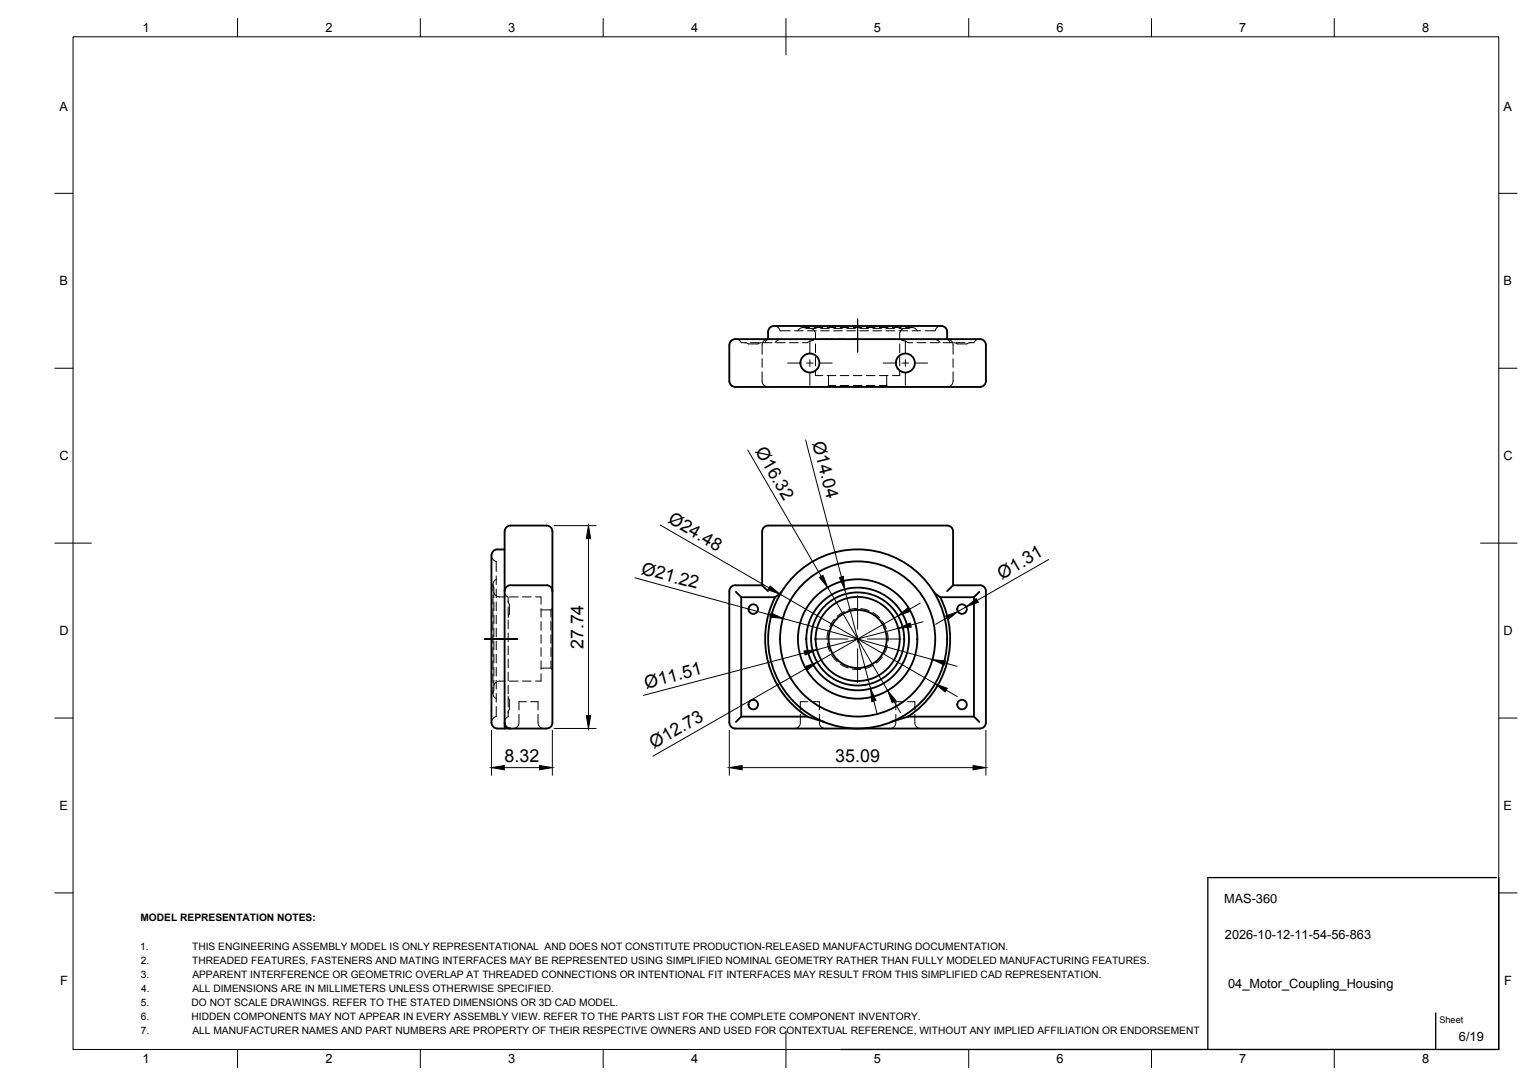
ISO-10303-21;
HEADER;
/* Generated by software containing ST-Developer
 * from STEP Tools, Inc. (www.steptools.com) 
 */

FILE_DESCRIPTION(
/* description */ (''),
/* implementation_level */ '2;1');

FILE_NAME(
/* name */ '04_Motor_Coupling_Housing.step',
/* time_stamp */ '2026-11-04T18:53:29-08:00',
/* author */ (''),
/* organization */ (''),
/* preprocessor_version */ 'ST-DEVELOPER v20.2',
/* originating_system */ 'Autodesk Translation Framework v15.17.0.0',
/* authorisation */ '');

FILE_SCHEMA (('AUTOMOTIVE_DESIGN { 1 0 10303 214 3 1 1 }'));
ENDSEC;

DATA;
#10=MECHANICAL_DESIGN_GEOMETRIC_PRESENTATION_REPRESENTATION('',(#1330),#100031);
#185=SPHERICAL_SURFACE('',#21262,0.800000000000001);
#186=SPHERICAL_SURFACE('',#21266,0.8);
#187=SPHERICAL_SURFACE('',#21275,0.800000000000001);
#188=SPHERICAL_SURFACE('',#21285,0.800000000000001);
#189=SPHERICAL_SURFACE('',#21292,0.800000000000003);
#190=SPHERICAL_SURFACE('',#21298,0.800000000000001);
#191=SPHERICAL_SURFACE('',#21302,0.800000000000001);
#192=SPHERICAL_SURFACE('',#21308,0.800000000000001);
#193=SPHERICAL_SURFACE('',#21315,0.8);
#194=SPHERICAL_SURFACE('',#21323,0.8);
#195=SPHERICAL_SURFACE('',#21330,0.8);
#196=SPHERICAL_SURFACE('',#21334,0.8);
#229=CONICAL_SURFACE('',#21430,4.075,0.785398163397448);
#662=CIRCLE('',#21263,0.800000000000001);
#663=CIRCLE('',#21264,0.800000000000001);
#664=CIRCLE('',#21265,0.800000000000001);
#665=CIRCLE('',#21267,0.800000000000001);
#666=CIRCLE('',#21268,0.8);
#667=CIRCLE('',#21269,0.800000000000001);
#668=CIRCLE('',#21271,0.800000000000001);
#669=CIRCLE('',#21273,0.8);
#670=CIRCLE('',#21276,0.800000000000001);
#671=CIRCLE('',#21277,0.800000000000001);
#672=CIRCLE('',#21278,0.800000000000001);
#673=CIRCLE('',#21280,0.800000000000001);
#674=CIRCLE('',#21286,0.800000000000001);
#675=CIRCLE('',#21287,0.800000000000001);
#676=CIRCLE('',#21288,0.800000000000001);
#677=CIRCLE('',#21291,0.800000000000001);
#678=CIRCLE('',#21293,0.800000000000001);
#679=CIRCLE('',#21294,0.800000000000003);
#680=CIRCLE('',#21295,0.800000000000001);
#681=CIRCLE('',#21299,0.800000000000001);
#682=CIRCLE('',#21300,0.800000000000001);
#683=CIRCLE('',#21301,0.800000000000001);
#684=CIRCLE('',#21303,0.8);
#685=CIRCLE('',#21304,0.800000000000001);
#686=CIRCLE('',#21305,0.800000000000001);
#687=CIRCLE('',#21307,0.8);
#688=CIRCLE('',#21309,0.800000000000001);
#689=CIRCLE('',#21310,0.800000000000001);
#690=CIRCLE('',#21311,0.800000000000001);
#691=CIRCLE('',#21316,0.799999999999998);
#692=CIRCLE('',#21317,0.799999999999997);
#693=CIRCLE('',#21318,0.799999999999999);
#694=CIRCLE('',#21322,0.800000000000001);
#695=CIRCLE('',#21324,0.799999999999999);
#696=CIRCLE('',#21325,0.800000000000001);
#697=CIRCLE('',#21328,0.800000000000001);
#698=CIRCLE('',#21331,0.799999999999999);
#699=CIRCLE('',#21332,12.24);
#700=CIRCLE('',#21333,12.24);
#701=CIRCLE('',#21335,0.800000000000001);
#702=CIRCLE('',#21338,2.1);
#703=CIRCLE('',#21339,2.1);
#704=CIRCLE('',#21350,5.7528);
#705=CIRCLE('',#21351,0.8);
#706=CIRCLE('',#21352,6.3648);
#707=CIRCLE('',#21354,5.7528);
#708=CIRCLE('',#21356,11.44);
#709=CIRCLE('',#21357,0.8);
#710=CIRCLE('',#21358,12.24);
#711=CIRCLE('',#21360,11.3943409947345);
#712=CIRCLE('',#21362,12.24);
#713=CIRCLE('',#21363,12.24);
#714=CIRCLE('',#21364,12.24);
#715=CIRCLE('',#21365,12.24);
#716=CIRCLE('',#21366,12.24);
#717=CIRCLE('',#21367,12.24);
#718=CIRCLE('',#21369,10.608);
#719=CIRCLE('',#21370,0.8);
#720=CIRCLE('',#21372,0.8);
#721=CIRCLE('',#21373,1.3);
#722=CIRCLE('',#21374,1.3);
#723=CIRCLE('',#21376,1.3);
#724=CIRCLE('',#21378,0.8);
#725=CIRCLE('',#21379,1.3);
#726=CIRCLE('',#21380,1.3);
#727=CIRCLE('',#21382,1.3);
#728=CIRCLE('',#21389,12.648);
#729=CIRCLE('',#21391,12.648);
#730=CIRCLE('',#21399,0.6528);
#731=CIRCLE('',#21400,0.8);
#732=CIRCLE('',#21401,1.13703729720046);
#733=CIRCLE('',#21403,1.13703729720046);
#734=CIRCLE('',#21405,0.6528);
#735=CIRCLE('',#21406,0.8);
#736=CIRCLE('',#21408,0.6528);
#737=CIRCLE('',#21409,0.8);
#738=CIRCLE('',#21410,1.13703729720046);
#739=CIRCLE('',#21412,1.13703729720046);
#740=CIRCLE('',#21414,0.6528);
#741=CIRCLE('',#21415,0.8);
#742=CIRCLE('',#21417,8.16);
#743=CIRCLE('',#21418,0.8);
#744=CIRCLE('',#21419,7.0176);
#745=CIRCLE('',#21429,3.975);
#746=CIRCLE('',#21431,3.975);
#747=CIRCLE('',#21432,4.175);
#1237=TOROIDAL_SURFACE('',#21349,6.5528,0.8);
#1238=TOROIDAL_SURFACE('',#21355,11.44,0.8);
#1239=TOROIDAL_SURFACE('',#21368,11.3943409947345,0.8);
#1240=TOROIDAL_SURFACE('',#21371,2.1,0.8);
#1241=TOROIDAL_SURFACE('',#21377,2.1,0.8);
#1242=TOROIDAL_SURFACE('',#21388,11.8802820935674,0.8);
#1243=TOROIDAL_SURFACE('',#21390,11.8802820935674,0.8);
#1244=TOROIDAL_SURFACE('',#21398,1.13703729720046,0.8);
#1245=TOROIDAL_SURFACE('',#21404,1.13703729720046,0.8);
#1246=TOROIDAL_SURFACE('',#21407,1.13703729720046,0.8);
#1247=TOROIDAL_SURFACE('',#21413,1.13703729720046,0.8);
#1248=TOROIDAL_SURFACE('',#21416,7.4416006562771,0.8);
#1294=SHAPE_REPRESENTATION_RELATIONSHIP('SRR','None',#100104,#1312);
#1312=ADVANCED_BREP_SHAPE_REPRESENTATION('',(#1348),#100016);
#1330=STYLED_ITEM('',(#100201),#1348);
#1348=MANIFOLD_SOLID_BREP('Body1',#20120);
#1455=PLANE('',#21336);
#1456=PLANE('',#21337);
#1457=PLANE('',#21340);
#1458=PLANE('',#21342);
#1459=PLANE('',#21343);
#1460=PLANE('',#21348);
#1461=PLANE('',#21359);
#1462=PLANE('',#21392);
#1463=PLANE('',#21402);
#1464=PLANE('',#21411);
#1465=PLANE('',#21420);
#1466=PLANE('',#21421);
#1467=PLANE('',#21422);
#1468=PLANE('',#21423);
#1469=PLANE('',#21424);
#1470=PLANE('',#21425);
#1471=PLANE('',#21426);
#1472=PLANE('',#21427);
#1473=PLANE('',#21428);
#1474=PLANE('',#21434);
#1475=PLANE('',#21435);
#1476=PLANE('',#21436);
#1743=FACE_BOUND('',#6778,.T.);
#1744=FACE_BOUND('',#6779,.T.);
#1745=FACE_BOUND('',#6792,.T.);
#1746=FACE_BOUND('',#6810,.T.);
#1747=FACE_BOUND('',#6811,.T.);
#1748=FACE_BOUND('',#6815,.T.);
#1749=FACE_BOUND('',#6816,.T.);
#1750=FACE_BOUND('',#6820,.T.);
#1751=FACE_BOUND('',#6828,.T.);
#1752=FACE_BOUND('',#6830,.T.);
#1753=FACE_BOUND('',#6834,.T.);
#1893=ELLIPSE('',#21282,1.13137084989848,0.8);
#1894=ELLIPSE('',#21284,1.13137084989848,0.8);
#1895=ELLIPSE('',#21314,1.13137084989848,0.8);
#1896=ELLIPSE('',#21346,1.13137084989848,0.8);
#1897=ELLIPSE('',#21384,1.13137084989848,0.800000000000001);
#1898=ELLIPSE('',#21385,1.13137084989848,0.800000000000001);
#1899=ELLIPSE('',#21394,1.13137084989848,0.8);
#1900=ELLIPSE('',#21396,1.13137084989848,0.799999999999998);
#2530=LINE('',#61146,#3817);
#2531=LINE('',#61147,#3818);
#2532=LINE('',#61152,#3819);
#2533=LINE('',#61153,#3820);
#2534=LINE('',#61155,#3821);
#2535=LINE('',#61156,#3822);
#2536=LINE('',#61167,#3823);
#2537=LINE('',#61168,#3824);
#2538=LINE('',#61171,#3825);
#2539=LINE('',#61173,#3826);
#2540=LINE('',#61177,#3827);
#2541=LINE('',#61179,#3828);
#2542=LINE('',#61189,#3829);
#2543=LINE('',#61190,#3830);
#2544=LINE('',#61195,#3831);
#2545=LINE('',#61196,#3832);
#2546=LINE('',#61205,#3833);
#2547=LINE('',#61206,#3834);
#2548=LINE('',#61208,#3835);
#2549=LINE('',#61209,#3836);
#2550=LINE('',#61228,#3837);
#2551=LINE('',#61229,#3838);
#2552=LINE('',#61238,#3839);
#2553=LINE('',#61239,#3840);
#2554=LINE('',#61242,#3841);
#2555=LINE('',#61244,#3842);
#2556=LINE('',#61254,#3843);
#2557=LINE('',#61255,#3844);
#2558=LINE('',#61257,#3845);
#2559=LINE('',#61258,#3846);
#2560=LINE('',#61263,#3847);
#2561=LINE('',#61264,#3848);
#2562=LINE('',#61270,#3849);
#2563=LINE('',#61271,#3850);
#2564=LINE('',#61275,#3851);
#2565=LINE('',#61276,#3852);
#2566=LINE('',#61278,#3853);
#2567=LINE('',#61279,#3854);
#2568=LINE('',#61389,#3855);
#2569=LINE('',#61391,#3856);
#2570=LINE('',#61397,#3857);
#2571=LINE('',#61399,#3858);
#2572=LINE('',#61403,#3859);
#2573=LINE('',#61406,#3860);
#2574=LINE('',#61409,#3861);
#2575=LINE('',#61411,#3862);
#2576=LINE('',#61412,#3863);
#2577=LINE('',#61414,#3864);
#2578=LINE('',#61424,#3865);
#2579=LINE('',#61436,#3866);
#2580=LINE('',#61459,#3867);
#2581=LINE('',#61469,#3868);
#2582=LINE('',#61474,#3869);
#2583=LINE('',#61478,#3870);
#2584=LINE('',#61496,#3871);
#2585=LINE('',#61497,#3872);
#2586=LINE('',#61516,#3873);
#2587=LINE('',#61517,#3874);
#2588=LINE('',#61558,#3875);
#2589=LINE('',#61560,#3876);
#2590=LINE('',#61561,#3877);
#2591=LINE('',#61565,#3878);
#2592=LINE('',#61568,#3879);
#2593=LINE('',#61571,#3880);
#2594=LINE('',#61619,#3881);
#2595=LINE('',#61622,#3882);
#3817=VECTOR('',#24951,10.);
#3818=VECTOR('',#24952,10.);
#3819=VECTOR('',#24957,10.);
#3820=VECTOR('',#24958,10.);
#3821=VECTOR('',#24961,10.);
#3822=VECTOR('',#24962,10.);
#3823=VECTOR('',#24975,10.);
#3824=VECTOR('',#24976,10.);
#3825=VECTOR('',#24979,10.);
#3826=VECTOR('',#24980,10.);
#3827=VECTOR('',#24985,10.);
#3828=VECTOR('',#24986,10.);
#3829=VECTOR('',#24999,10.);
#3830=VECTOR('',#25000,10.);
#3831=VECTOR('',#25005,10.);
#3832=VECTOR('',#25006,10.);
#3833=VECTOR('',#25017,10.);
#3834=VECTOR('',#25018,10.);
#3835=VECTOR('',#25021,10.);
#3836=VECTOR('',#25022,10.);
#3837=VECTOR('',#25043,10.);
#3838=VECTOR('',#25044,10.);
#3839=VECTOR('',#25055,10.);
#3840=VECTOR('',#25056,10.);
#3841=VECTOR('',#25059,10.);
#3842=VECTOR('',#25060,10.);
#3843=VECTOR('',#25073,10.);
#3844=VECTOR('',#25074,10.);
#3845=VECTOR('',#25077,10.);
#3846=VECTOR('',#25078,10.);
#3847=VECTOR('',#25083,10.);
#3848=VECTOR('',#25084,10.);
#3849=VECTOR('',#25093,10.);
#3850=VECTOR('',#25094,10.);
#3851=VECTOR('',#25099,10.);
#3852=VECTOR('',#25100,10.);
#3853=VECTOR('',#25103,10.);
#3854=VECTOR('',#25104,10.);
#3855=VECTOR('',#25119,10.);
#3856=VECTOR('',#25122,10.);
#3857=VECTOR('',#25129,10.);
#3858=VECTOR('',#25132,10.);
#3859=VECTOR('',#25139,10.);
#3860=VECTOR('',#25142,10.);
#3861=VECTOR('',#25145,10.);
#3862=VECTOR('',#25148,10.);
#3863=VECTOR('',#25149,10.);
#3864=VECTOR('',#25152,10.);
#3865=VECTOR('',#25165,5.7528);
#3866=VECTOR('',#25180,12.24);
#3867=VECTOR('',#25209,1.3);
#3868=VECTOR('',#25222,1.3);
#3869=VECTOR('',#25227,0.8);
#3870=VECTOR('',#25230,10.);
#3871=VECTOR('',#25235,10.);
#3872=VECTOR('',#25236,0.8);
#3873=VECTOR('',#25239,0.8);
#3874=VECTOR('',#25240,10.);
#3875=VECTOR('',#25251,10.);
#3876=VECTOR('',#25252,0.8);
#3877=VECTOR('',#25253,10.);
#3878=VECTOR('',#25258,10.);
#3879=VECTOR('',#25261,10.);
#3880=VECTOR('',#25266,10.);
#3881=VECTOR('',#25335,4.075);
#3882=VECTOR('',#25340,3.975);
#4767=CYLINDRICAL_SURFACE('',#21270,0.8);
#4768=CYLINDRICAL_SURFACE('',#21272,0.8);
#4769=CYLINDRICAL_SURFACE('',#21274,0.8);
#4770=CYLINDRICAL_SURFACE('',#21279,0.8);
#4771=CYLINDRICAL_SURFACE('',#21281,0.8);
#4772=CYLINDRICAL_SURFACE('',#21283,0.8);
#4773=CYLINDRICAL_SURFACE('',#21289,0.8);
#4774=CYLINDRICAL_SURFACE('',#21290,0.8);
#4775=CYLINDRICAL_SURFACE('',#21296,0.8);
#4776=CYLINDRICAL_SURFACE('',#21297,0.8);
#4777=CYLINDRICAL_SURFACE('',#21306,0.8);
#4778=CYLINDRICAL_SURFACE('',#21312,0.8);
#4779=CYLINDRICAL_SURFACE('',#21313,0.8);
#4780=CYLINDRICAL_SURFACE('',#21319,0.8);
#4781=CYLINDRICAL_SURFACE('',#21320,0.8);
#4782=CYLINDRICAL_SURFACE('',#21321,0.8);
#4783=CYLINDRICAL_SURFACE('',#21326,0.8);
#4784=CYLINDRICAL_SURFACE('',#21327,0.8);
#4785=CYLINDRICAL_SURFACE('',#21329,0.8);
#4786=CYLINDRICAL_SURFACE('',#21341,0.8);
#4787=CYLINDRICAL_SURFACE('',#21344,0.8);
#4788=CYLINDRICAL_SURFACE('',#21345,0.8);
#4789=CYLINDRICAL_SURFACE('',#21347,0.8);
#4790=CYLINDRICAL_SURFACE('',#21353,5.7528);
#4791=CYLINDRICAL_SURFACE('',#21361,12.24);
#4792=CYLINDRICAL_SURFACE('',#21375,1.3);
#4793=CYLINDRICAL_SURFACE('',#21381,1.3);
#4794=CYLINDRICAL_SURFACE('',#21383,0.8);
#4795=CYLINDRICAL_SURFACE('',#21386,0.8);
#4796=CYLINDRICAL_SURFACE('',#21387,0.799999999999998);
#4797=CYLINDRICAL_SURFACE('',#21393,0.8);
#4798=CYLINDRICAL_SURFACE('',#21395,0.799999999999998);
#4799=CYLINDRICAL_SURFACE('',#21397,0.8);
#4800=CYLINDRICAL_SURFACE('',#21433,3.975);
#5537=FACE_OUTER_BOUND('',#6743,.T.);
#5538=FACE_OUTER_BOUND('',#6744,.T.);
#5539=FACE_OUTER_BOUND('',#6745,.T.);
#5540=FACE_OUTER_BOUND('',#6746,.T.);
#5541=FACE_OUTER_BOUND('',#6747,.T.);
#5542=FACE_OUTER_BOUND('',#6748,.T.);
#5543=FACE_OUTER_BOUND('',#6749,.T.);
#5544=FACE_OUTER_BOUND('',#6750,.T.);
#5545=FACE_OUTER_BOUND('',#6751,.T.);
#5546=FACE_OUTER_BOUND('',#6752,.T.);
#5547=FACE_OUTER_BOUND('',#6753,.T.);
#5548=FACE_OUTER_BOUND('',#6754,.T.);
#5549=FACE_OUTER_BOUND('',#6755,.T.);
#5550=FACE_OUTER_BOUND('',#6756,.T.);
#5551=FACE_OUTER_BOUND('',#6757,.T.);
#5552=FACE_OUTER_BOUND('',#6758,.T.);
#5553=FACE_OUTER_BOUND('',#6759,.T.);
#5554=FACE_OUTER_BOUND('',#6760,.T.);
#5555=FACE_OUTER_BOUND('',#6761,.T.);
#5556=FACE_OUTER_BOUND('',#6762,.T.);
#5557=FACE_OUTER_BOUND('',#6763,.T.);
#5558=FACE_OUTER_BOUND('',#6764,.T.);
#5559=FACE_OUTER_BOUND('',#6765,.T.);
#5560=FACE_OUTER_BOUND('',#6766,.T.);
#5561=FACE_OUTER_BOUND('',#6767,.T.);
#5562=FACE_OUTER_BOUND('',#6768,.T.);
#5563=FACE_OUTER_BOUND('',#6769,.T.);
#5564=FACE_OUTER_BOUND('',#6770,.T.);
#5565=FACE_OUTER_BOUND('',#6771,.T.);
#5566=FACE_OUTER_BOUND('',#6772,.T.);
#5567=FACE_OUTER_BOUND('',#6773,.T.);
#5568=FACE_OUTER_BOUND('',#6774,.T.);
#5569=FACE_OUTER_BOUND('',#6775,.T.);
#5570=FACE_OUTER_BOUND('',#6776,.T.);
#5571=FACE_OUTER_BOUND('',#6777,.T.);
#5572=FACE_OUTER_BOUND('',#6780,.T.);
#5573=FACE_OUTER_BOUND('',#6781,.T.);
#5574=FACE_OUTER_BOUND('',#6782,.T.);
#5575=FACE_OUTER_BOUND('',#6783,.T.);
#5576=FACE_OUTER_BOUND('',#6784,.T.);
#5577=FACE_OUTER_BOUND('',#6785,.T.);
#5578=FACE_OUTER_BOUND('',#6786,.T.);
#5579=FACE_OUTER_BOUND('',#6787,.T.);
#5580=FACE_OUTER_BOUND('',#6788,.T.);
#5581=FACE_OUTER_BOUND('',#6789,.T.);
#5582=FACE_OUTER_BOUND('',#6790,.T.);
#5583=FACE_OUTER_BOUND('',#6791,.T.);
#5584=FACE_OUTER_BOUND('',#6793,.T.);
#5585=FACE_OUTER_BOUND('',#6794,.T.);
#5586=FACE_OUTER_BOUND('',#6795,.T.);
#5587=FACE_OUTER_BOUND('',#6796,.T.);
#5588=FACE_OUTER_BOUND('',#6797,.T.);
#5589=FACE_OUTER_BOUND('',#6798,.T.);
#5590=FACE_OUTER_BOUND('',#6799,.T.);
#5591=FACE_OUTER_BOUND('',#6800,.T.);
#5592=FACE_OUTER_BOUND('',#6801,.T.);
#5593=FACE_OUTER_BOUND('',#6802,.T.);
#5594=FACE_OUTER_BOUND('',#6803,.T.);
#5595=FACE_OUTER_BOUND('',#6804,.T.);
#5596=FACE_OUTER_BOUND('',#6805,.T.);
#5597=FACE_OUTER_BOUND('',#6806,.T.);
#5598=FACE_OUTER_BOUND('',#6807,.T.);
#5599=FACE_OUTER_BOUND('',#6808,.T.);
#5600=FACE_OUTER_BOUND('',#6809,.T.);
#5601=FACE_OUTER_BOUND('',#6812,.T.);
#5602=FACE_OUTER_BOUND('',#6813,.T.);
#5603=FACE_OUTER_BOUND('',#6814,.T.);
#5604=FACE_OUTER_BOUND('',#6817,.T.);
#5605=FACE_OUTER_BOUND('',#6818,.T.);
#5606=FACE_OUTER_BOUND('',#6819,.T.);
#5607=FACE_OUTER_BOUND('',#6821,.T.);
#5608=FACE_OUTER_BOUND('',#6822,.T.);
#5609=FACE_OUTER_BOUND('',#6823,.T.);
#5610=FACE_OUTER_BOUND('',#6824,.T.);
#5611=FACE_OUTER_BOUND('',#6825,.T.);
#5612=FACE_OUTER_BOUND('',#6826,.T.);
#5613=FACE_OUTER_BOUND('',#6827,.T.);
#5614=FACE_OUTER_BOUND('',#6829,.T.);
#5615=FACE_OUTER_BOUND('',#6831,.T.);
#5616=FACE_OUTER_BOUND('',#6832,.T.);
#5617=FACE_OUTER_BOUND('',#6833,.T.);
#5618=FACE_OUTER_BOUND('',#6835,.T.);
#5619=FACE_OUTER_BOUND('',#6836,.T.);
#6743=EDGE_LOOP('',(#15455,#15456,#15457));
#6744=EDGE_LOOP('',(#15458,#15459,#15460));
#6745=EDGE_LOOP('',(#15461,#15462,#15463,#15464));
#6746=EDGE_LOOP('',(#15465,#15466,#15467,#15468));
#6747=EDGE_LOOP('',(#15469,#15470,#15471,#15472));
#6748=EDGE_LOOP('',(#15473,#15474,#15475));
#6749=EDGE_LOOP('',(#15476,#15477,#15478,#15479));
#6750=EDGE_LOOP('',(#15480,#15481,#15482,#15483));
#6751=EDGE_LOOP('',(#15484,#15485,#15486,#15487));
#6752=EDGE_LOOP('',(#15488,#15489,#15490));
#6753=EDGE_LOOP('',(#15491,#15492,#15493,#15494));
#6754=EDGE_LOOP('',(#15495,#15496,#15497,#15498));
#6755=EDGE_LOOP('',(#15499,#15500,#15501));
#6756=EDGE_LOOP('',(#15502,#15503,#15504,#15505));
#6757=EDGE_LOOP('',(#15506,#15507,#15508,#15509));
#6758=EDGE_LOOP('',(#15510,#15511,#15512));
#6759=EDGE_LOOP('',(#15513,#15514,#15515));
#6760=EDGE_LOOP('',(#15516,#15517,#15518,#15519));
#6761=EDGE_LOOP('',(#15520,#15521,#15522));
#6762=EDGE_LOOP('',(#15523,#15524,#15525,#15526));
#6763=EDGE_LOOP('',(#15527,#15528,#15529,#15530));
#6764=EDGE_LOOP('',(#15531,#15532,#15533));
#6765=EDGE_LOOP('',(#15534,#15535,#15536,#15537));
#6766=EDGE_LOOP('',(#15538,#15539,#15540,#15541));
#6767=EDGE_LOOP('',(#15542,#15543,#15544,#15545));
#6768=EDGE_LOOP('',(#15546,#15547,#15548));
#6769=EDGE_LOOP('',(#15549,#15550,#15551,#15552));
#6770=EDGE_LOOP('',(#15553,#15554,#15555,#15556));
#6771=EDGE_LOOP('',(#15557,#15558,#15559,#15560));
#6772=EDGE_LOOP('',(#15561,#15562,#15563,#15564));
#6773=EDGE_LOOP('',(#15565,#15566,#15567));
#6774=EDGE_LOOP('',(#15568,#15569,#15570,#15571));
#6775=EDGE_LOOP('',(#15572,#15573,#15574));
#6776=EDGE_LOOP('',(#15575,#15576,#15577,#15578));
#6777=EDGE_LOOP('',(#15579,#15580,#15581,#15582,#15583,#15584,#15585));
#6778=EDGE_LOOP('',(#15586));
#6779=EDGE_LOOP('',(#15587));
#6780=EDGE_LOOP('',(#15588,#15589,#15590,#15591));
#6781=EDGE_LOOP('',(#15592,#15593,#15594,#15595));
#6782=EDGE_LOOP('',(#15596,#15597,#15598,#15599));
#6783=EDGE_LOOP('',(#15600,#15601,#15602,#15603));
#6784=EDGE_LOOP('',(#15604,#15605,#15606,#15607));
#6785=EDGE_LOOP('',(#15608,#15609,#15610,#15611));
#6786=EDGE_LOOP('',(#15612,#15613,#15614,#15615));
#6787=EDGE_LOOP('',(#15616,#15617,#15618,#15619));
#6788=EDGE_LOOP('',(#15620,#15621,#15622,#15623));
#6789=EDGE_LOOP('',(#15624,#15625,#15626,#15627));
#6790=EDGE_LOOP('',(#15628,#15629,#15630,#15631));
#6791=EDGE_LOOP('',(#15632));
#6792=EDGE_LOOP('',(#15633));
#6793=EDGE_LOOP('',(#15634,#15635,#15636,#15637,#15638,#15639,#15640,#15641,
#15642,#15643,#15644,#15645,#15646));
#6794=EDGE_LOOP('',(#15647,#15648,#15649,#15650));
#6795=EDGE_LOOP('',(#15651,#15652,#15653,#15654,#15655));
#6796=EDGE_LOOP('',(#15656,#15657,#15658,#15659,#15660));
#6797=EDGE_LOOP('',(#15661,#15662,#15663,#15664,#15665));
#6798=EDGE_LOOP('',(#15666,#15667,#15668,#15669,#15670));
#6799=EDGE_LOOP('',(#15671,#15672,#15673,#15674));
#6800=EDGE_LOOP('',(#15675,#15676,#15677,#15678));
#6801=EDGE_LOOP('',(#15679,#15680,#15681,#15682));
#6802=EDGE_LOOP('',(#15683,#15684,#15685,#15686,#15687));
#6803=EDGE_LOOP('',(#15688,#15689,#15690,#15691));
#6804=EDGE_LOOP('',(#15692,#15693,#15694,#15695,#15696,#15697,#15698,#15699,
#15700,#15701,#15702,#15703,#15704,#15705,#15706,#15707,#15708,#15709));
#6805=EDGE_LOOP('',(#15710,#15711,#15712,#15713));
#6806=EDGE_LOOP('',(#15714,#15715,#15716,#15717));
#6807=EDGE_LOOP('',(#15718,#15719,#15720,#15721));
#6808=EDGE_LOOP('',(#15722,#15723,#15724,#15725));
#6809=EDGE_LOOP('',(#15726,#15727,#15728,#15729));
#6810=EDGE_LOOP('',(#15730));
#6811=EDGE_LOOP('',(#15731));
#6812=EDGE_LOOP('',(#15732,#15733,#15734,#15735));
#6813=EDGE_LOOP('',(#15736,#15737,#15738,#15739));
#6814=EDGE_LOOP('',(#15740,#15741,#15742,#15743));
#6815=EDGE_LOOP('',(#15744));
#6816=EDGE_LOOP('',(#15745));
#6817=EDGE_LOOP('',(#15746,#15747,#15748,#15749));
#6818=EDGE_LOOP('',(#15750,#15751,#15752,#15753));
#6819=EDGE_LOOP('',(#15754));
#6820=EDGE_LOOP('',(#15755));
#6821=EDGE_LOOP('',(#15756));
#6822=EDGE_LOOP('',(#15757));
#6823=EDGE_LOOP('',(#15758));
#6824=EDGE_LOOP('',(#15759));
#6825=EDGE_LOOP('',(#15760));
#6826=EDGE_LOOP('',(#15761));
#6827=EDGE_LOOP('',(#15762));
#6828=EDGE_LOOP('',(#15763));
#6829=EDGE_LOOP('',(#15764));
#6830=EDGE_LOOP('',(#15765));
#6831=EDGE_LOOP('',(#15766,#15767,#15768,#15769));
#6832=EDGE_LOOP('',(#15770,#15771,#15772,#15773));
#6833=EDGE_LOOP('',(#15774,#15775,#15776,#15777,#15778,#15779,#15780,#15781));
#6834=EDGE_LOOP('',(#15782));
#6835=EDGE_LOOP('',(#15783,#15784,#15785,#15786));
#6836=EDGE_LOOP('',(#15787,#15788,#15789,#15790));
#7691=B_SPLINE_CURVE_WITH_KNOTS('',3,(#61321,#61322,#61323,#61324,#61325,
#61326,#61327,#61328),.UNSPECIFIED.,.F.,.F.,(4,1,1,2,4),(0.886448358529016,
0.974711394590892,1.06297443065277,1.3277635388384,1.32899011332275),
 .UNSPECIFIED.);
#7692=B_SPLINE_CURVE_WITH_KNOTS('',3,(#61330,#61331,#61332,#61333),
 .UNSPECIFIED.,.F.,.F.,(4,4),(-0.111726598224603,-0.107341152681297),
 .UNSPECIFIED.);
#7693=B_SPLINE_CURVE_WITH_KNOTS('',3,(#61334,#61335,#61336,#61337,#61338,
#61339,#61340,#61341,#61342,#61343,#61344),.UNSPECIFIED.,.F.,.F.,(4,1,2,
2,2,4),(-0.107341152681297,-0.0558632991123017,0.,0.110861644323643,0.224510220235513,
0.333435958612223),.UNSPECIFIED.);
#7694=B_SPLINE_CURVE_WITH_KNOTS('',3,(#61380,#61381,#61382,#61383,#61384,
#61385),.UNSPECIFIED.,.F.,.F.,(4,2,4),(-0.00122657448435937,0.,0.44131518030938),
 .UNSPECIFIED.);
#7695=B_SPLINE_CURVE_WITH_KNOTS('',3,(#61482,#61483,#61484,#61485,#61486,
#61487,#61488,#61489,#61490,#61491,#61492,#61493,#61494,#61495),
 .UNSPECIFIED.,.F.,.F.,(4,2,2,2,2,2,4),(-4.00267101076923,-3.97980879370467,
-3.86999664917252,-3.77335331431691,-3.71746622872759,-3.69720180919271,
-3.6853266531919),.UNSPECIFIED.);
#7696=B_SPLINE_CURVE_WITH_KNOTS('',3,(#61500,#61501,#61502,#61503,#61504,
#61505,#61506,#61507,#61508,#61509,#61510,#61511,#61512,#61513,#61514,#61515),
 .UNSPECIFIED.,.F.,.F.,(4,2,2,2,2,2,2,4),(-0.827425542979679,-0.826220339571657,
-0.824592036045519,-0.820443574755297,-0.781909027879826,-0.745118942396318,
-0.725073379095867,-0.724859868833872),.UNSPECIFIED.);
#7697=B_SPLINE_CURVE_WITH_KNOTS('',3,(#61522,#61523,#61524,#61525,#61526,
#61527,#61528,#61529,#61530,#61531,#61532,#61533,#61534,#61535),
 .UNSPECIFIED.,.F.,.F.,(4,2,2,2,2,2,4),(0.0275854854772956,0.0545477001455191,
0.147140622467183,0.269392757315554,0.297346368764049,0.310172163976987,
0.314080909465034),.UNSPECIFIED.);
#7698=B_SPLINE_CURVE_WITH_KNOTS('',3,(#61538,#61539,#61540,#61541,#61542,
#61543,#61544,#61545,#61546,#61547,#61548,#61549,#61550,#61551,#61552,#61553,
#61554,#61555),.UNSPECIFIED.,.F.,.F.,(4,2,2,2,2,2,2,2,4),(0.121304483487225,
0.121522867409781,0.122956741161004,0.125266692582563,0.133381651141487,
0.155840009541048,0.198528123526881,0.228063475003939,0.232050075067381),
 .UNSPECIFIED.);
#8819=VERTEX_POINT('',#61129);
#8820=VERTEX_POINT('',#61130);
#8821=VERTEX_POINT('',#61132);
#8822=VERTEX_POINT('',#61136);
#8823=VERTEX_POINT('',#61137);
#8824=VERTEX_POINT('',#61139);
#8825=VERTEX_POINT('',#61143);
#8826=VERTEX_POINT('',#61144);
#8827=VERTEX_POINT('',#61149);
#8828=VERTEX_POINT('',#61150);
#8829=VERTEX_POINT('',#61158);
#8830=VERTEX_POINT('',#61159);
#8831=VERTEX_POINT('',#61161);
#8832=VERTEX_POINT('',#61165);
#8833=VERTEX_POINT('',#61170);
#8834=VERTEX_POINT('',#61172);
#8835=VERTEX_POINT('',#61176);
#8836=VERTEX_POINT('',#61178);
#8837=VERTEX_POINT('',#61182);
#8838=VERTEX_POINT('',#61183);
#8839=VERTEX_POINT('',#61185);
#8840=VERTEX_POINT('',#61192);
#8841=VERTEX_POINT('',#61193);
#8842=VERTEX_POINT('',#61198);
#8843=VERTEX_POINT('',#61199);
#8844=VERTEX_POINT('',#61201);
#8845=VERTEX_POINT('',#61211);
#8846=VERTEX_POINT('',#61212);
#8847=VERTEX_POINT('',#61214);
#8848=VERTEX_POINT('',#61218);
#8849=VERTEX_POINT('',#61219);
#8850=VERTEX_POINT('',#61221);
#8851=VERTEX_POINT('',#61225);
#8852=VERTEX_POINT('',#61226);
#8853=VERTEX_POINT('',#61231);
#8854=VERTEX_POINT('',#61232);
#8855=VERTEX_POINT('',#61234);
#8856=VERTEX_POINT('',#61241);
#8857=VERTEX_POINT('',#61243);
#8858=VERTEX_POINT('',#61247);
#8859=VERTEX_POINT('',#61248);
#8860=VERTEX_POINT('',#61250);
#8861=VERTEX_POINT('',#61260);
#8862=VERTEX_POINT('',#61261);
#8863=VERTEX_POINT('',#61266);
#8864=VERTEX_POINT('',#61273);
#8865=VERTEX_POINT('',#61320);
#8866=VERTEX_POINT('',#61329);
#8867=VERTEX_POINT('',#61377);
#8868=VERTEX_POINT('',#61392);
#8869=VERTEX_POINT('',#61394);
#8870=VERTEX_POINT('',#61405);
#8871=VERTEX_POINT('',#61407);
#8872=VERTEX_POINT('',#61416);
#8873=VERTEX_POINT('',#61418);
#8874=VERTEX_POINT('',#61422);
#8875=VERTEX_POINT('',#61426);
#8876=VERTEX_POINT('',#61428);
#8877=VERTEX_POINT('',#61432);
#8878=VERTEX_POINT('',#61435);
#8879=VERTEX_POINT('',#61437);
#8880=VERTEX_POINT('',#61440);
#8881=VERTEX_POINT('',#61442);
#8882=VERTEX_POINT('',#61444);
#8883=VERTEX_POINT('',#61448);
#8884=VERTEX_POINT('',#61452);
#8885=VERTEX_POINT('',#61454);
#8886=VERTEX_POINT('',#61458);
#8887=VERTEX_POINT('',#61462);
#8888=VERTEX_POINT('',#61464);
#8889=VERTEX_POINT('',#61468);
#8890=VERTEX_POINT('',#61472);
#8891=VERTEX_POINT('',#61473);
#8892=VERTEX_POINT('',#61475);
#8893=VERTEX_POINT('',#61477);
#8894=VERTEX_POINT('',#61481);
#8895=VERTEX_POINT('',#61499);
#8896=VERTEX_POINT('',#61521);
#8897=VERTEX_POINT('',#61536);
#8898=VERTEX_POINT('',#61557);
#8899=VERTEX_POINT('',#61559);
#8900=VERTEX_POINT('',#61563);
#8901=VERTEX_POINT('',#61567);
#8902=VERTEX_POINT('',#61573);
#8903=VERTEX_POINT('',#61575);
#8904=VERTEX_POINT('',#61579);
#8905=VERTEX_POINT('',#61582);
#8906=VERTEX_POINT('',#61586);
#8907=VERTEX_POINT('',#61588);
#8908=VERTEX_POINT('',#61592);
#8909=VERTEX_POINT('',#61595);
#8910=VERTEX_POINT('',#61599);
#8911=VERTEX_POINT('',#61601);
#8912=VERTEX_POINT('',#61613);
#8913=VERTEX_POINT('',#61616);
#8914=VERTEX_POINT('',#61618);
#11202=EDGE_CURVE('',#8819,#8820,#662,.F.);
#11203=EDGE_CURVE('',#8821,#8819,#663,.F.);
#11204=EDGE_CURVE('',#8820,#8821,#664,.F.);
#11205=EDGE_CURVE('',#8822,#8823,#665,.F.);
#11206=EDGE_CURVE('',#8824,#8822,#666,.F.);
#11207=EDGE_CURVE('',#8823,#8824,#667,.F.);
#11208=EDGE_CURVE('',#8825,#8826,#668,.T.);
#11209=EDGE_CURVE('',#8826,#8824,#2530,.T.);
#11210=EDGE_CURVE('',#8822,#8825,#2531,.T.);
#11211=EDGE_CURVE('',#8827,#8828,#669,.T.);
#11212=EDGE_CURVE('',#8828,#8823,#2532,.T.);
#11213=EDGE_CURVE('',#8824,#8827,#2533,.T.);
#11214=EDGE_CURVE('',#8819,#8822,#2534,.T.);
#11215=EDGE_CURVE('',#8823,#8821,#2535,.T.);
#11216=EDGE_CURVE('',#8829,#8830,#670,.F.);
#11217=EDGE_CURVE('',#8831,#8829,#671,.F.);
#11218=EDGE_CURVE('',#8830,#8831,#672,.F.);
#11219=EDGE_CURVE('',#8828,#8832,#673,.T.);
#11220=EDGE_CURVE('',#8832,#8831,#2536,.T.);
#11221=EDGE_CURVE('',#8829,#8828,#2537,.T.);
#11222=EDGE_CURVE('',#8833,#8830,#2538,.T.);
#11223=EDGE_CURVE('',#8831,#8834,#2539,.T.);
#11224=EDGE_CURVE('',#8834,#8833,#1893,.T.);
#11225=EDGE_CURVE('',#8835,#8819,#2540,.T.);
#11226=EDGE_CURVE('',#8820,#8836,#2541,.T.);
#11227=EDGE_CURVE('',#8836,#8835,#1894,.T.);
#11228=EDGE_CURVE('',#8837,#8838,#674,.F.);
#11229=EDGE_CURVE('',#8839,#8837,#675,.F.);
#11230=EDGE_CURVE('',#8838,#8839,#676,.F.);
#11231=EDGE_CURVE('',#8834,#8839,#2542,.T.);
#11232=EDGE_CURVE('',#8837,#8833,#2543,.T.);
#11233=EDGE_CURVE('',#8840,#8841,#677,.T.);
#11234=EDGE_CURVE('',#8841,#8838,#2544,.T.);
#11235=EDGE_CURVE('',#8839,#8840,#2545,.T.);
#11236=EDGE_CURVE('',#8842,#8843,#678,.F.);
#11237=EDGE_CURVE('',#8844,#8842,#679,.F.);
#11238=EDGE_CURVE('',#8843,#8844,#680,.F.);
#11239=EDGE_CURVE('',#8836,#8844,#2546,.T.);
#11240=EDGE_CURVE('',#8842,#8835,#2547,.T.);
#11241=EDGE_CURVE('',#8838,#8843,#2548,.T.);
#11242=EDGE_CURVE('',#8844,#8837,#2549,.T.);
#11243=EDGE_CURVE('',#8845,#8846,#681,.F.);
#11244=EDGE_CURVE('',#8847,#8845,#682,.F.);
#11245=EDGE_CURVE('',#8846,#8847,#683,.F.);
#11246=EDGE_CURVE('',#8848,#8849,#684,.F.);
#11247=EDGE_CURVE('',#8850,#8848,#685,.F.);
#11248=EDGE_CURVE('',#8849,#8850,#686,.F.);
#11249=EDGE_CURVE('',#8851,#8852,#687,.T.);
#11250=EDGE_CURVE('',#8852,#8850,#2550,.T.);
#11251=EDGE_CURVE('',#8848,#8851,#2551,.T.);
#11252=EDGE_CURVE('',#8853,#8854,#688,.F.);
#11253=EDGE_CURVE('',#8855,#8853,#689,.F.);
#11254=EDGE_CURVE('',#8854,#8855,#690,.F.);
#11255=EDGE_CURVE('',#8853,#8849,#2552,.T.);
#11256=EDGE_CURVE('',#8850,#8855,#2553,.T.);
#11257=EDGE_CURVE('',#8856,#8854,#2554,.T.);
#11258=EDGE_CURVE('',#8855,#8857,#2555,.T.);
#11259=EDGE_CURVE('',#8857,#8856,#1895,.T.);
#11260=EDGE_CURVE('',#8858,#8859,#691,.T.);
#11261=EDGE_CURVE('',#8859,#8860,#692,.T.);
#11262=EDGE_CURVE('',#8860,#8858,#693,.T.);
#11263=EDGE_CURVE('',#8858,#8853,#2556,.T.);
#11264=EDGE_CURVE('',#8854,#8859,#2557,.T.);
#11265=EDGE_CURVE('',#8857,#8847,#2558,.T.);
#11266=EDGE_CURVE('',#8845,#8856,#2559,.T.);
#11267=EDGE_CURVE('',#8861,#8862,#694,.T.);
#11268=EDGE_CURVE('',#8862,#8848,#2560,.T.);
#11269=EDGE_CURVE('',#8849,#8861,#2561,.T.);
#11270=EDGE_CURVE('',#8861,#8863,#695,.T.);
#11271=EDGE_CURVE('',#8863,#8862,#696,.T.);
#11272=EDGE_CURVE('',#8843,#8846,#2562,.T.);
#11273=EDGE_CURVE('',#8847,#8842,#2563,.T.);
#11274=EDGE_CURVE('',#8841,#8864,#697,.T.);
#11275=EDGE_CURVE('',#8864,#8845,#2564,.T.);
#11276=EDGE_CURVE('',#8846,#8841,#2565,.T.);
#11277=EDGE_CURVE('',#8830,#8820,#2566,.T.);
#11278=EDGE_CURVE('',#8821,#8829,#2567,.T.);
#11279=EDGE_CURVE('',#8851,#8865,#7691,.T.);
#11280=EDGE_CURVE('',#8865,#8866,#7692,.T.);
#11281=EDGE_CURVE('',#8866,#8852,#7693,.T.);
#11282=EDGE_CURVE('',#8840,#8864,#698,.T.);
#11283=EDGE_CURVE('',#8825,#8867,#699,.T.);
#11284=EDGE_CURVE('',#8867,#8865,#700,.T.);
#11285=EDGE_CURVE('',#8865,#8826,#7694,.T.);
#11286=EDGE_CURVE('',#8827,#8832,#701,.T.);
#11287=EDGE_CURVE('',#8833,#8836,#2568,.T.);
#11288=EDGE_CURVE('',#8827,#8862,#2569,.T.);
#11289=EDGE_CURVE('',#8868,#8868,#702,.T.);
#11290=EDGE_CURVE('',#8869,#8869,#703,.T.);
#11291=EDGE_CURVE('',#8861,#8858,#2570,.T.);
#11292=EDGE_CURVE('',#8860,#8863,#2571,.T.);
#11293=EDGE_CURVE('',#8863,#8832,#2572,.T.);
#11294=EDGE_CURVE('',#8859,#8870,#2573,.T.);
#11295=EDGE_CURVE('',#8870,#8871,#1896,.T.);
#11296=EDGE_CURVE('',#8871,#8860,#2574,.T.);
#11297=EDGE_CURVE('',#8840,#8871,#2575,.T.);
#11298=EDGE_CURVE('',#8870,#8864,#2576,.T.);
#11299=EDGE_CURVE('',#8856,#8870,#2577,.T.);
#11300=EDGE_CURVE('',#8872,#8872,#704,.T.);
#11301=EDGE_CURVE('',#8872,#8873,#705,.T.);
#11302=EDGE_CURVE('',#8873,#8873,#706,.T.);
#11303=EDGE_CURVE('',#8874,#8874,#707,.T.);
#11304=EDGE_CURVE('',#8874,#8872,#2578,.T.);
#11305=EDGE_CURVE('',#8875,#8875,#708,.T.);
#11306=EDGE_CURVE('',#8875,#8876,#709,.T.);
#11307=EDGE_CURVE('',#8876,#8876,#710,.T.);
#11308=EDGE_CURVE('',#8877,#8877,#711,.T.);
#11309=EDGE_CURVE('',#8876,#8878,#2579,.T.);
#11310=EDGE_CURVE('',#8879,#8878,#712,.T.);
#11311=EDGE_CURVE('',#8852,#8879,#713,.T.);
#11312=EDGE_CURVE('',#8880,#8825,#714,.T.);
#11313=EDGE_CURVE('',#8881,#8880,#715,.T.);
#11314=EDGE_CURVE('',#8882,#8881,#716,.T.);
#11315=EDGE_CURVE('',#8878,#8882,#717,.T.);
#11316=EDGE_CURVE('',#8883,#8883,#718,.T.);
#11317=EDGE_CURVE('',#8883,#8877,#719,.T.);
#11318=EDGE_CURVE('',#8869,#8884,#720,.T.);
#11319=EDGE_CURVE('',#8884,#8885,#721,.T.);
#11320=EDGE_CURVE('',#8885,#8884,#722,.T.);
#11321=EDGE_CURVE('',#8885,#8886,#2580,.T.);
#11322=EDGE_CURVE('',#8886,#8886,#723,.T.);
#11323=EDGE_CURVE('',#8868,#8887,#724,.T.);
#11324=EDGE_CURVE('',#8887,#8888,#725,.T.);
#11325=EDGE_CURVE('',#8888,#8887,#726,.T.);
#11326=EDGE_CURVE('',#8888,#8889,#2581,.T.);
#11327=EDGE_CURVE('',#8889,#8889,#727,.T.);
#11328=EDGE_CURVE('',#8890,#8891,#2582,.T.);
#11329=EDGE_CURVE('',#8891,#8892,#1897,.T.);
#11330=EDGE_CURVE('',#8892,#8893,#2583,.T.);
#11331=EDGE_CURVE('',#8893,#8890,#1898,.T.);
#11332=EDGE_CURVE('',#8879,#8894,#7695,.F.);
#11333=EDGE_CURVE('',#8894,#8892,#2584,.T.);
#11334=EDGE_CURVE('',#8891,#8879,#2585,.T.);
#11335=EDGE_CURVE('',#8882,#8895,#7696,.T.);
#11336=EDGE_CURVE('',#8882,#8890,#2586,.T.);
#11337=EDGE_CURVE('',#8893,#8895,#2587,.T.);
#11338=EDGE_CURVE('',#8895,#8894,#728,.T.);
#11339=EDGE_CURVE('',#8880,#8896,#7697,.F.);
#11340=EDGE_CURVE('',#8896,#8897,#729,.T.);
#11341=EDGE_CURVE('',#8881,#8897,#7698,.T.);
#11342=EDGE_CURVE('',#8898,#8881,#2588,.T.);
#11343=EDGE_CURVE('',#8899,#8898,#2589,.T.);
#11344=EDGE_CURVE('',#8880,#8899,#2590,.T.);
#11345=EDGE_CURVE('',#8899,#8900,#1899,.T.);
#11346=EDGE_CURVE('',#8900,#8896,#2591,.T.);
#11347=EDGE_CURVE('',#8897,#8901,#2592,.T.);
#11348=EDGE_CURVE('',#8901,#8898,#1900,.T.);
#11349=EDGE_CURVE('',#8901,#8900,#2593,.T.);
#11350=EDGE_CURVE('',#8902,#8902,#730,.T.);
#11351=EDGE_CURVE('',#8902,#8903,#731,.T.);
#11352=EDGE_CURVE('',#8903,#8903,#732,.T.);
#11353=EDGE_CURVE('',#8904,#8904,#733,.T.);
#11354=EDGE_CURVE('',#8905,#8905,#734,.T.);
#11355=EDGE_CURVE('',#8905,#8904,#735,.T.);
#11356=EDGE_CURVE('',#8906,#8906,#736,.T.);
#11357=EDGE_CURVE('',#8906,#8907,#737,.T.);
#11358=EDGE_CURVE('',#8907,#8907,#738,.T.);
#11359=EDGE_CURVE('',#8908,#8908,#739,.T.);
#11360=EDGE_CURVE('',#8909,#8909,#740,.T.);
#11361=EDGE_CURVE('',#8909,#8908,#741,.T.);
#11362=EDGE_CURVE('',#8910,#8910,#742,.T.);
#11363=EDGE_CURVE('',#8910,#8911,#743,.T.);
#11364=EDGE_CURVE('',#8911,#8911,#744,.T.);
#11365=EDGE_CURVE('',#8912,#8912,#745,.T.);
#11366=EDGE_CURVE('',#8913,#8913,#746,.T.);
#11367=EDGE_CURVE('',#8913,#8914,#2594,.T.);
#11368=EDGE_CURVE('',#8914,#8914,#747,.T.);
#11369=EDGE_CURVE('',#8913,#8912,#2595,.T.);
#15455=ORIENTED_EDGE('',*,*,#11202,.F.);
#15456=ORIENTED_EDGE('',*,*,#11203,.F.);
#15457=ORIENTED_EDGE('',*,*,#11204,.F.);
#15458=ORIENTED_EDGE('',*,*,#11205,.F.);
#15459=ORIENTED_EDGE('',*,*,#11206,.F.);
#15460=ORIENTED_EDGE('',*,*,#11207,.F.);
#15461=ORIENTED_EDGE('',*,*,#11208,.T.);
#15462=ORIENTED_EDGE('',*,*,#11209,.T.);
#15463=ORIENTED_EDGE('',*,*,#11206,.T.);
#15464=ORIENTED_EDGE('',*,*,#11210,.T.);
#15465=ORIENTED_EDGE('',*,*,#11211,.T.);
#15466=ORIENTED_EDGE('',*,*,#11212,.T.);
#15467=ORIENTED_EDGE('',*,*,#11207,.T.);
#15468=ORIENTED_EDGE('',*,*,#11213,.T.);
#15469=ORIENTED_EDGE('',*,*,#11203,.T.);
#15470=ORIENTED_EDGE('',*,*,#11214,.T.);
#15471=ORIENTED_EDGE('',*,*,#11205,.T.);
#15472=ORIENTED_EDGE('',*,*,#11215,.T.);
#15473=ORIENTED_EDGE('',*,*,#11216,.F.);
#15474=ORIENTED_EDGE('',*,*,#11217,.F.);
#15475=ORIENTED_EDGE('',*,*,#11218,.F.);
#15476=ORIENTED_EDGE('',*,*,#11219,.T.);
#15477=ORIENTED_EDGE('',*,*,#11220,.T.);
#15478=ORIENTED_EDGE('',*,*,#11217,.T.);
#15479=ORIENTED_EDGE('',*,*,#11221,.T.);
#15480=ORIENTED_EDGE('',*,*,#11222,.T.);
#15481=ORIENTED_EDGE('',*,*,#11218,.T.);
#15482=ORIENTED_EDGE('',*,*,#11223,.T.);
#15483=ORIENTED_EDGE('',*,*,#11224,.T.);
#15484=ORIENTED_EDGE('',*,*,#11225,.T.);
#15485=ORIENTED_EDGE('',*,*,#11202,.T.);
#15486=ORIENTED_EDGE('',*,*,#11226,.T.);
#15487=ORIENTED_EDGE('',*,*,#11227,.T.);
#15488=ORIENTED_EDGE('',*,*,#11228,.F.);
#15489=ORIENTED_EDGE('',*,*,#11229,.F.);
#15490=ORIENTED_EDGE('',*,*,#11230,.F.);
#15491=ORIENTED_EDGE('',*,*,#11231,.T.);
#15492=ORIENTED_EDGE('',*,*,#11229,.T.);
#15493=ORIENTED_EDGE('',*,*,#11232,.T.);
#15494=ORIENTED_EDGE('',*,*,#11224,.F.);
#15495=ORIENTED_EDGE('',*,*,#11233,.T.);
#15496=ORIENTED_EDGE('',*,*,#11234,.T.);
#15497=ORIENTED_EDGE('',*,*,#11230,.T.);
#15498=ORIENTED_EDGE('',*,*,#11235,.T.);
#15499=ORIENTED_EDGE('',*,*,#11236,.F.);
#15500=ORIENTED_EDGE('',*,*,#11237,.F.);
#15501=ORIENTED_EDGE('',*,*,#11238,.F.);
#15502=ORIENTED_EDGE('',*,*,#11239,.T.);
#15503=ORIENTED_EDGE('',*,*,#11237,.T.);
#15504=ORIENTED_EDGE('',*,*,#11240,.T.);
#15505=ORIENTED_EDGE('',*,*,#11227,.F.);
#15506=ORIENTED_EDGE('',*,*,#11228,.T.);
#15507=ORIENTED_EDGE('',*,*,#11241,.T.);
#15508=ORIENTED_EDGE('',*,*,#11238,.T.);
#15509=ORIENTED_EDGE('',*,*,#11242,.T.);
#15510=ORIENTED_EDGE('',*,*,#11243,.F.);
#15511=ORIENTED_EDGE('',*,*,#11244,.F.);
#15512=ORIENTED_EDGE('',*,*,#11245,.F.);
#15513=ORIENTED_EDGE('',*,*,#11246,.F.);
#15514=ORIENTED_EDGE('',*,*,#11247,.F.);
#15515=ORIENTED_EDGE('',*,*,#11248,.F.);
#15516=ORIENTED_EDGE('',*,*,#11249,.T.);
#15517=ORIENTED_EDGE('',*,*,#11250,.T.);
#15518=ORIENTED_EDGE('',*,*,#11247,.T.);
#15519=ORIENTED_EDGE('',*,*,#11251,.T.);
#15520=ORIENTED_EDGE('',*,*,#11252,.F.);
#15521=ORIENTED_EDGE('',*,*,#11253,.F.);
#15522=ORIENTED_EDGE('',*,*,#11254,.F.);
#15523=ORIENTED_EDGE('',*,*,#11253,.T.);
#15524=ORIENTED_EDGE('',*,*,#11255,.T.);
#15525=ORIENTED_EDGE('',*,*,#11248,.T.);
#15526=ORIENTED_EDGE('',*,*,#11256,.T.);
#15527=ORIENTED_EDGE('',*,*,#11257,.T.);
#15528=ORIENTED_EDGE('',*,*,#11254,.T.);
#15529=ORIENTED_EDGE('',*,*,#11258,.T.);
#15530=ORIENTED_EDGE('',*,*,#11259,.T.);
#15531=ORIENTED_EDGE('',*,*,#11260,.T.);
#15532=ORIENTED_EDGE('',*,*,#11261,.T.);
#15533=ORIENTED_EDGE('',*,*,#11262,.T.);
#15534=ORIENTED_EDGE('',*,*,#11260,.F.);
#15535=ORIENTED_EDGE('',*,*,#11263,.T.);
#15536=ORIENTED_EDGE('',*,*,#11252,.T.);
#15537=ORIENTED_EDGE('',*,*,#11264,.T.);
#15538=ORIENTED_EDGE('',*,*,#11265,.T.);
#15539=ORIENTED_EDGE('',*,*,#11244,.T.);
#15540=ORIENTED_EDGE('',*,*,#11266,.T.);
#15541=ORIENTED_EDGE('',*,*,#11259,.F.);
#15542=ORIENTED_EDGE('',*,*,#11267,.T.);
#15543=ORIENTED_EDGE('',*,*,#11268,.T.);
#15544=ORIENTED_EDGE('',*,*,#11246,.T.);
#15545=ORIENTED_EDGE('',*,*,#11269,.T.);
#15546=ORIENTED_EDGE('',*,*,#11267,.F.);
#15547=ORIENTED_EDGE('',*,*,#11270,.T.);
#15548=ORIENTED_EDGE('',*,*,#11271,.T.);
#15549=ORIENTED_EDGE('',*,*,#11236,.T.);
#15550=ORIENTED_EDGE('',*,*,#11272,.T.);
#15551=ORIENTED_EDGE('',*,*,#11245,.T.);
#15552=ORIENTED_EDGE('',*,*,#11273,.T.);
#15553=ORIENTED_EDGE('',*,*,#11274,.T.);
#15554=ORIENTED_EDGE('',*,*,#11275,.T.);
#15555=ORIENTED_EDGE('',*,*,#11243,.T.);
#15556=ORIENTED_EDGE('',*,*,#11276,.T.);
#15557=ORIENTED_EDGE('',*,*,#11216,.T.);
#15558=ORIENTED_EDGE('',*,*,#11277,.T.);
#15559=ORIENTED_EDGE('',*,*,#11204,.T.);
#15560=ORIENTED_EDGE('',*,*,#11278,.T.);
#15561=ORIENTED_EDGE('',*,*,#11249,.F.);
#15562=ORIENTED_EDGE('',*,*,#11279,.T.);
#15563=ORIENTED_EDGE('',*,*,#11280,.T.);
#15564=ORIENTED_EDGE('',*,*,#11281,.T.);
#15565=ORIENTED_EDGE('',*,*,#11233,.F.);
#15566=ORIENTED_EDGE('',*,*,#11282,.T.);
#15567=ORIENTED_EDGE('',*,*,#11274,.F.);
#15568=ORIENTED_EDGE('',*,*,#11208,.F.);
#15569=ORIENTED_EDGE('',*,*,#11283,.T.);
#15570=ORIENTED_EDGE('',*,*,#11284,.T.);
#15571=ORIENTED_EDGE('',*,*,#11285,.T.);
#15572=ORIENTED_EDGE('',*,*,#11211,.F.);
#15573=ORIENTED_EDGE('',*,*,#11286,.T.);
#15574=ORIENTED_EDGE('',*,*,#11219,.F.);
#15575=ORIENTED_EDGE('',*,*,#11232,.F.);
#15576=ORIENTED_EDGE('',*,*,#11242,.F.);
#15577=ORIENTED_EDGE('',*,*,#11239,.F.);
#15578=ORIENTED_EDGE('',*,*,#11287,.F.);
#15579=ORIENTED_EDGE('',*,*,#11213,.F.);
#15580=ORIENTED_EDGE('',*,*,#11209,.F.);
#15581=ORIENTED_EDGE('',*,*,#11285,.F.);
#15582=ORIENTED_EDGE('',*,*,#11279,.F.);
#15583=ORIENTED_EDGE('',*,*,#11251,.F.);
#15584=ORIENTED_EDGE('',*,*,#11268,.F.);
#15585=ORIENTED_EDGE('',*,*,#11288,.F.);
#15586=ORIENTED_EDGE('',*,*,#11289,.F.);
#15587=ORIENTED_EDGE('',*,*,#11290,.F.);
#15588=ORIENTED_EDGE('',*,*,#11269,.F.);
#15589=ORIENTED_EDGE('',*,*,#11255,.F.);
#15590=ORIENTED_EDGE('',*,*,#11263,.F.);
#15591=ORIENTED_EDGE('',*,*,#11291,.F.);
#15592=ORIENTED_EDGE('',*,*,#11270,.F.);
#15593=ORIENTED_EDGE('',*,*,#11291,.T.);
#15594=ORIENTED_EDGE('',*,*,#11262,.F.);
#15595=ORIENTED_EDGE('',*,*,#11292,.T.);
#15596=ORIENTED_EDGE('',*,*,#11212,.F.);
#15597=ORIENTED_EDGE('',*,*,#11221,.F.);
#15598=ORIENTED_EDGE('',*,*,#11278,.F.);
#15599=ORIENTED_EDGE('',*,*,#11215,.F.);
#15600=ORIENTED_EDGE('',*,*,#11234,.F.);
#15601=ORIENTED_EDGE('',*,*,#11276,.F.);
#15602=ORIENTED_EDGE('',*,*,#11272,.F.);
#15603=ORIENTED_EDGE('',*,*,#11241,.F.);
#15604=ORIENTED_EDGE('',*,*,#11286,.F.);
#15605=ORIENTED_EDGE('',*,*,#11288,.T.);
#15606=ORIENTED_EDGE('',*,*,#11271,.F.);
#15607=ORIENTED_EDGE('',*,*,#11293,.T.);
#15608=ORIENTED_EDGE('',*,*,#11261,.F.);
#15609=ORIENTED_EDGE('',*,*,#11294,.T.);
#15610=ORIENTED_EDGE('',*,*,#11295,.T.);
#15611=ORIENTED_EDGE('',*,*,#11296,.T.);
#15612=ORIENTED_EDGE('',*,*,#11282,.F.);
#15613=ORIENTED_EDGE('',*,*,#11297,.T.);
#15614=ORIENTED_EDGE('',*,*,#11295,.F.);
#15615=ORIENTED_EDGE('',*,*,#11298,.T.);
#15616=ORIENTED_EDGE('',*,*,#11257,.F.);
#15617=ORIENTED_EDGE('',*,*,#11299,.T.);
#15618=ORIENTED_EDGE('',*,*,#11294,.F.);
#15619=ORIENTED_EDGE('',*,*,#11264,.F.);
#15620=ORIENTED_EDGE('',*,*,#11300,.T.);
#15621=ORIENTED_EDGE('',*,*,#11301,.T.);
#15622=ORIENTED_EDGE('',*,*,#11302,.T.);
#15623=ORIENTED_EDGE('',*,*,#11301,.F.);
#15624=ORIENTED_EDGE('',*,*,#11303,.F.);
#15625=ORIENTED_EDGE('',*,*,#11304,.T.);
#15626=ORIENTED_EDGE('',*,*,#11300,.F.);
#15627=ORIENTED_EDGE('',*,*,#11304,.F.);
#15628=ORIENTED_EDGE('',*,*,#11305,.T.);
#15629=ORIENTED_EDGE('',*,*,#11306,.T.);
#15630=ORIENTED_EDGE('',*,*,#11307,.T.);
#15631=ORIENTED_EDGE('',*,*,#11306,.F.);
#15632=ORIENTED_EDGE('',*,*,#11305,.F.);
#15633=ORIENTED_EDGE('',*,*,#11308,.F.);
#15634=ORIENTED_EDGE('',*,*,#11307,.F.);
#15635=ORIENTED_EDGE('',*,*,#11309,.T.);
#15636=ORIENTED_EDGE('',*,*,#11310,.F.);
#15637=ORIENTED_EDGE('',*,*,#11311,.F.);
#15638=ORIENTED_EDGE('',*,*,#11281,.F.);
#15639=ORIENTED_EDGE('',*,*,#11280,.F.);
#15640=ORIENTED_EDGE('',*,*,#11284,.F.);
#15641=ORIENTED_EDGE('',*,*,#11283,.F.);
#15642=ORIENTED_EDGE('',*,*,#11312,.F.);
#15643=ORIENTED_EDGE('',*,*,#11313,.F.);
#15644=ORIENTED_EDGE('',*,*,#11314,.F.);
#15645=ORIENTED_EDGE('',*,*,#11315,.F.);
#15646=ORIENTED_EDGE('',*,*,#11309,.F.);
#15647=ORIENTED_EDGE('',*,*,#11316,.T.);
#15648=ORIENTED_EDGE('',*,*,#11317,.T.);
#15649=ORIENTED_EDGE('',*,*,#11308,.T.);
#15650=ORIENTED_EDGE('',*,*,#11317,.F.);
#15651=ORIENTED_EDGE('',*,*,#11290,.T.);
#15652=ORIENTED_EDGE('',*,*,#11318,.T.);
#15653=ORIENTED_EDGE('',*,*,#11319,.T.);
#15654=ORIENTED_EDGE('',*,*,#11320,.T.);
#15655=ORIENTED_EDGE('',*,*,#11318,.F.);
#15656=ORIENTED_EDGE('',*,*,#11320,.F.);
#15657=ORIENTED_EDGE('',*,*,#11321,.T.);
#15658=ORIENTED_EDGE('',*,*,#11322,.T.);
#15659=ORIENTED_EDGE('',*,*,#11321,.F.);
#15660=ORIENTED_EDGE('',*,*,#11319,.F.);
#15661=ORIENTED_EDGE('',*,*,#11289,.T.);
#15662=ORIENTED_EDGE('',*,*,#11323,.T.);
#15663=ORIENTED_EDGE('',*,*,#11324,.T.);
#15664=ORIENTED_EDGE('',*,*,#11325,.T.);
#15665=ORIENTED_EDGE('',*,*,#11323,.F.);
#15666=ORIENTED_EDGE('',*,*,#11325,.F.);
#15667=ORIENTED_EDGE('',*,*,#11326,.T.);
#15668=ORIENTED_EDGE('',*,*,#11327,.T.);
#15669=ORIENTED_EDGE('',*,*,#11326,.F.);
#15670=ORIENTED_EDGE('',*,*,#11324,.F.);
#15671=ORIENTED_EDGE('',*,*,#11328,.T.);
#15672=ORIENTED_EDGE('',*,*,#11329,.T.);
#15673=ORIENTED_EDGE('',*,*,#11330,.T.);
#15674=ORIENTED_EDGE('',*,*,#11331,.T.);
#15675=ORIENTED_EDGE('',*,*,#11332,.T.);
#15676=ORIENTED_EDGE('',*,*,#11333,.T.);
#15677=ORIENTED_EDGE('',*,*,#11329,.F.);
#15678=ORIENTED_EDGE('',*,*,#11334,.T.);
#15679=ORIENTED_EDGE('',*,*,#11335,.F.);
#15680=ORIENTED_EDGE('',*,*,#11336,.T.);
#15681=ORIENTED_EDGE('',*,*,#11331,.F.);
#15682=ORIENTED_EDGE('',*,*,#11337,.T.);
#15683=ORIENTED_EDGE('',*,*,#11310,.T.);
#15684=ORIENTED_EDGE('',*,*,#11315,.T.);
#15685=ORIENTED_EDGE('',*,*,#11335,.T.);
#15686=ORIENTED_EDGE('',*,*,#11338,.T.);
#15687=ORIENTED_EDGE('',*,*,#11332,.F.);
#15688=ORIENTED_EDGE('',*,*,#11339,.T.);
#15689=ORIENTED_EDGE('',*,*,#11340,.T.);
#15690=ORIENTED_EDGE('',*,*,#11341,.F.);
#15691=ORIENTED_EDGE('',*,*,#11313,.T.);
#15692=ORIENTED_EDGE('',*,*,#11250,.F.);
#15693=ORIENTED_EDGE('',*,*,#11311,.T.);
#15694=ORIENTED_EDGE('',*,*,#11334,.F.);
#15695=ORIENTED_EDGE('',*,*,#11328,.F.);
#15696=ORIENTED_EDGE('',*,*,#11336,.F.);
#15697=ORIENTED_EDGE('',*,*,#11314,.T.);
#15698=ORIENTED_EDGE('',*,*,#11342,.F.);
#15699=ORIENTED_EDGE('',*,*,#11343,.F.);
#15700=ORIENTED_EDGE('',*,*,#11344,.F.);
#15701=ORIENTED_EDGE('',*,*,#11312,.T.);
#15702=ORIENTED_EDGE('',*,*,#11210,.F.);
#15703=ORIENTED_EDGE('',*,*,#11214,.F.);
#15704=ORIENTED_EDGE('',*,*,#11225,.F.);
#15705=ORIENTED_EDGE('',*,*,#11240,.F.);
#15706=ORIENTED_EDGE('',*,*,#11273,.F.);
#15707=ORIENTED_EDGE('',*,*,#11265,.F.);
#15708=ORIENTED_EDGE('',*,*,#11258,.F.);
#15709=ORIENTED_EDGE('',*,*,#11256,.F.);
#15710=ORIENTED_EDGE('',*,*,#11344,.T.);
#15711=ORIENTED_EDGE('',*,*,#11345,.T.);
#15712=ORIENTED_EDGE('',*,*,#11346,.T.);
#15713=ORIENTED_EDGE('',*,*,#11339,.F.);
#15714=ORIENTED_EDGE('',*,*,#11347,.T.);
#15715=ORIENTED_EDGE('',*,*,#11348,.T.);
#15716=ORIENTED_EDGE('',*,*,#11342,.T.);
#15717=ORIENTED_EDGE('',*,*,#11341,.T.);
#15718=ORIENTED_EDGE('',*,*,#11343,.T.);
#15719=ORIENTED_EDGE('',*,*,#11348,.F.);
#15720=ORIENTED_EDGE('',*,*,#11349,.T.);
#15721=ORIENTED_EDGE('',*,*,#11345,.F.);
#15722=ORIENTED_EDGE('',*,*,#11350,.T.);
#15723=ORIENTED_EDGE('',*,*,#11351,.T.);
#15724=ORIENTED_EDGE('',*,*,#11352,.T.);
#15725=ORIENTED_EDGE('',*,*,#11351,.F.);
#15726=ORIENTED_EDGE('',*,*,#11337,.F.);
#15727=ORIENTED_EDGE('',*,*,#11330,.F.);
#15728=ORIENTED_EDGE('',*,*,#11333,.F.);
#15729=ORIENTED_EDGE('',*,*,#11338,.F.);
#15730=ORIENTED_EDGE('',*,*,#11353,.F.);
#15731=ORIENTED_EDGE('',*,*,#11352,.F.);
#15732=ORIENTED_EDGE('',*,*,#11354,.T.);
#15733=ORIENTED_EDGE('',*,*,#11355,.T.);
#15734=ORIENTED_EDGE('',*,*,#11353,.T.);
#15735=ORIENTED_EDGE('',*,*,#11355,.F.);
#15736=ORIENTED_EDGE('',*,*,#11356,.T.);
#15737=ORIENTED_EDGE('',*,*,#11357,.T.);
#15738=ORIENTED_EDGE('',*,*,#11358,.T.);
#15739=ORIENTED_EDGE('',*,*,#11357,.F.);
#15740=ORIENTED_EDGE('',*,*,#11349,.F.);
#15741=ORIENTED_EDGE('',*,*,#11347,.F.);
#15742=ORIENTED_EDGE('',*,*,#11340,.F.);
#15743=ORIENTED_EDGE('',*,*,#11346,.F.);
#15744=ORIENTED_EDGE('',*,*,#11359,.F.);
#15745=ORIENTED_EDGE('',*,*,#11358,.F.);
#15746=ORIENTED_EDGE('',*,*,#11360,.T.);
#15747=ORIENTED_EDGE('',*,*,#11361,.T.);
#15748=ORIENTED_EDGE('',*,*,#11359,.T.);
#15749=ORIENTED_EDGE('',*,*,#11361,.F.);
#15750=ORIENTED_EDGE('',*,*,#11362,.T.);
#15751=ORIENTED_EDGE('',*,*,#11363,.T.);
#15752=ORIENTED_EDGE('',*,*,#11364,.T.);
#15753=ORIENTED_EDGE('',*,*,#11363,.F.);
#15754=ORIENTED_EDGE('',*,*,#11364,.F.);
#15755=ORIENTED_EDGE('',*,*,#11302,.F.);
#15756=ORIENTED_EDGE('',*,*,#11360,.F.);
#15757=ORIENTED_EDGE('',*,*,#11356,.F.);
#15758=ORIENTED_EDGE('',*,*,#11354,.F.);
#15759=ORIENTED_EDGE('',*,*,#11350,.F.);
#15760=ORIENTED_EDGE('',*,*,#11327,.F.);
#15761=ORIENTED_EDGE('',*,*,#11322,.F.);
#15762=ORIENTED_EDGE('',*,*,#11316,.F.);
#15763=ORIENTED_EDGE('',*,*,#11362,.F.);
#15764=ORIENTED_EDGE('',*,*,#11303,.T.);
#15765=ORIENTED_EDGE('',*,*,#11365,.F.);
#15766=ORIENTED_EDGE('',*,*,#11366,.T.);
#15767=ORIENTED_EDGE('',*,*,#11367,.T.);
#15768=ORIENTED_EDGE('',*,*,#11368,.T.);
#15769=ORIENTED_EDGE('',*,*,#11367,.F.);
#15770=ORIENTED_EDGE('',*,*,#11366,.F.);
#15771=ORIENTED_EDGE('',*,*,#11369,.T.);
#15772=ORIENTED_EDGE('',*,*,#11365,.T.);
#15773=ORIENTED_EDGE('',*,*,#11369,.F.);
#15774=ORIENTED_EDGE('',*,*,#11220,.F.);
#15775=ORIENTED_EDGE('',*,*,#11293,.F.);
#15776=ORIENTED_EDGE('',*,*,#11292,.F.);
#15777=ORIENTED_EDGE('',*,*,#11296,.F.);
#15778=ORIENTED_EDGE('',*,*,#11297,.F.);
#15779=ORIENTED_EDGE('',*,*,#11235,.F.);
#15780=ORIENTED_EDGE('',*,*,#11231,.F.);
#15781=ORIENTED_EDGE('',*,*,#11223,.F.);
#15782=ORIENTED_EDGE('',*,*,#11368,.F.);
#15783=ORIENTED_EDGE('',*,*,#11275,.F.);
#15784=ORIENTED_EDGE('',*,*,#11298,.F.);
#15785=ORIENTED_EDGE('',*,*,#11299,.F.);
#15786=ORIENTED_EDGE('',*,*,#11266,.F.);
#15787=ORIENTED_EDGE('',*,*,#11222,.F.);
#15788=ORIENTED_EDGE('',*,*,#11287,.T.);
#15789=ORIENTED_EDGE('',*,*,#11226,.F.);
#15790=ORIENTED_EDGE('',*,*,#11277,.F.);
#18931=B_SPLINE_SURFACE_WITH_KNOTS('',3,3,((#61280,#61281,#61282,#61283,
#61284,#61285,#61286,#61287),(#61288,#61289,#61290,#61291,#61292,#61293,
#61294,#61295),(#61296,#61297,#61298,#61299,#61300,#61301,#61302,#61303),
(#61304,#61305,#61306,#61307,#61308,#61309,#61310,#61311),(#61312,#61313,
#61314,#61315,#61316,#61317,#61318,#61319)),.UNSPECIFIED.,.F.,.F.,.F.,(4,
1,4),(4,2,1,1,4),(-0.00184352937430784,0.571428571428571,1.),(-1.32899011332275,
-1.3277635388384,-1.06297443065277,-0.974711394590892,-0.884839152512737),
 .UNSPECIFIED.);
#18932=B_SPLINE_SURFACE_WITH_KNOTS('',3,3,((#61347,#61348,#61349,#61350,
#61351,#61352),(#61353,#61354,#61355,#61356,#61357,#61358),(#61359,#61360,
#61361,#61362,#61363,#61364),(#61365,#61366,#61367,#61368,#61369,#61370),
(#61371,#61372,#61373,#61374,#61375,#61376)),.UNSPECIFIED.,.F.,.F.,.F.,
(4,1,4),(4,2,4),(-0.0048972902445563,0.571428571428571,1.),(-0.446212470553937,
0.,0.00122657448435937),.UNSPECIFIED.);
#19471=ADVANCED_FACE('',(#5537),#185,.T.);
#19472=ADVANCED_FACE('',(#5538),#186,.T.);
#19473=ADVANCED_FACE('',(#5539),#4767,.T.);
#19474=ADVANCED_FACE('',(#5540),#4768,.T.);
#19475=ADVANCED_FACE('',(#5541),#4769,.T.);
#19476=ADVANCED_FACE('',(#5542),#187,.T.);
#19477=ADVANCED_FACE('',(#5543),#4770,.T.);
#19478=ADVANCED_FACE('',(#5544),#4771,.T.);
#19479=ADVANCED_FACE('',(#5545),#4772,.T.);
#19480=ADVANCED_FACE('',(#5546),#188,.T.);
#19481=ADVANCED_FACE('',(#5547),#4773,.T.);
#19482=ADVANCED_FACE('',(#5548),#4774,.T.);
#19483=ADVANCED_FACE('',(#5549),#189,.T.);
#19484=ADVANCED_FACE('',(#5550),#4775,.T.);
#19485=ADVANCED_FACE('',(#5551),#4776,.T.);
#19486=ADVANCED_FACE('',(#5552),#190,.T.);
#19487=ADVANCED_FACE('',(#5553),#191,.T.);
#19488=ADVANCED_FACE('',(#5554),#4777,.T.);
#19489=ADVANCED_FACE('',(#5555),#192,.T.);
#19490=ADVANCED_FACE('',(#5556),#4778,.T.);
#19491=ADVANCED_FACE('',(#5557),#4779,.T.);
#19492=ADVANCED_FACE('',(#5558),#193,.T.);
#19493=ADVANCED_FACE('',(#5559),#4780,.T.);
#19494=ADVANCED_FACE('',(#5560),#4781,.T.);
#19495=ADVANCED_FACE('',(#5561),#4782,.T.);
#19496=ADVANCED_FACE('',(#5562),#194,.T.);
#19497=ADVANCED_FACE('',(#5563),#4783,.T.);
#19498=ADVANCED_FACE('',(#5564),#4784,.T.);
#19499=ADVANCED_FACE('',(#5565),#4785,.T.);
#19500=ADVANCED_FACE('',(#5566),#18931,.F.);
#19501=ADVANCED_FACE('',(#5567),#195,.T.);
#19502=ADVANCED_FACE('',(#5568),#18932,.F.);
#19503=ADVANCED_FACE('',(#5569),#196,.T.);
#19504=ADVANCED_FACE('',(#5570),#1455,.T.);
#19505=ADVANCED_FACE('',(#5571,#1743,#1744),#1456,.F.);
#19506=ADVANCED_FACE('',(#5572),#1457,.T.);
#19507=ADVANCED_FACE('',(#5573),#4786,.T.);
#19508=ADVANCED_FACE('',(#5574),#1458,.T.);
#19509=ADVANCED_FACE('',(#5575),#1459,.T.);
#19510=ADVANCED_FACE('',(#5576),#4787,.T.);
#19511=ADVANCED_FACE('',(#5577),#4788,.T.);
#19512=ADVANCED_FACE('',(#5578),#4789,.T.);
#19513=ADVANCED_FACE('',(#5579),#1460,.T.);
#19514=ADVANCED_FACE('',(#5580),#1237,.T.);
#19515=ADVANCED_FACE('',(#5581),#4790,.F.);
#19516=ADVANCED_FACE('',(#5582),#1238,.T.);
#19517=ADVANCED_FACE('',(#5583,#1745),#1461,.T.);
#19518=ADVANCED_FACE('',(#5584),#4791,.T.);
#19519=ADVANCED_FACE('',(#5585),#1239,.T.);
#19520=ADVANCED_FACE('',(#5586),#1240,.T.);
#19521=ADVANCED_FACE('',(#5587),#4792,.F.);
#19522=ADVANCED_FACE('',(#5588),#1241,.T.);
#19523=ADVANCED_FACE('',(#5589),#4793,.F.);
#19524=ADVANCED_FACE('',(#5590),#4794,.T.);
#19525=ADVANCED_FACE('',(#5591),#4795,.T.);
#19526=ADVANCED_FACE('',(#5592),#4796,.T.);
#19527=ADVANCED_FACE('',(#5593),#1242,.T.);
#19528=ADVANCED_FACE('',(#5594),#1243,.T.);
#19529=ADVANCED_FACE('',(#5595),#1462,.T.);
#19530=ADVANCED_FACE('',(#5596),#4797,.T.);
#19531=ADVANCED_FACE('',(#5597),#4798,.T.);
#19532=ADVANCED_FACE('',(#5598),#4799,.T.);
#19533=ADVANCED_FACE('',(#5599),#1244,.T.);
#19534=ADVANCED_FACE('',(#5600,#1746,#1747),#1463,.T.);
#19535=ADVANCED_FACE('',(#5601),#1245,.T.);
#19536=ADVANCED_FACE('',(#5602),#1246,.T.);
#19537=ADVANCED_FACE('',(#5603,#1748,#1749),#1464,.T.);
#19538=ADVANCED_FACE('',(#5604),#1247,.T.);
#19539=ADVANCED_FACE('',(#5605),#1248,.T.);
#19540=ADVANCED_FACE('',(#5606,#1750),#1465,.T.);
#19541=ADVANCED_FACE('',(#5607),#1466,.T.);
#19542=ADVANCED_FACE('',(#5608),#1467,.T.);
#19543=ADVANCED_FACE('',(#5609),#1468,.T.);
#19544=ADVANCED_FACE('',(#5610),#1469,.T.);
#19545=ADVANCED_FACE('',(#5611),#1470,.F.);
#19546=ADVANCED_FACE('',(#5612),#1471,.F.);
#19547=ADVANCED_FACE('',(#5613,#1751),#1472,.T.);
#19548=ADVANCED_FACE('',(#5614,#1752),#1473,.T.);
#19549=ADVANCED_FACE('',(#5615),#229,.F.);
#19550=ADVANCED_FACE('',(#5616),#4800,.F.);
#19551=ADVANCED_FACE('',(#5617,#1753),#1474,.T.);
#19552=ADVANCED_FACE('',(#5618),#1475,.T.);
#19553=ADVANCED_FACE('',(#5619),#1476,.T.);
#20120=CLOSED_SHELL('',(#19471,#19472,#19473,#19474,#19475,#19476,#19477,
#19478,#19479,#19480,#19481,#19482,#19483,#19484,#19485,#19486,#19487,#19488,
#19489,#19490,#19491,#19492,#19493,#19494,#19495,#19496,#19497,#19498,#19499,
#19500,#19501,#19502,#19503,#19504,#19505,#19506,#19507,#19508,#19509,#19510,
#19511,#19512,#19513,#19514,#19515,#19516,#19517,#19518,#19519,#19520,#19521,
#19522,#19523,#19524,#19525,#19526,#19527,#19528,#19529,#19530,#19531,#19532,
#19533,#19534,#19535,#19536,#19537,#19538,#19539,#19540,#19541,#19542,#19543,
#19544,#19545,#19546,#19547,#19548,#19549,#19550,#19551,#19552,#19553));
#21261=AXIS2_PLACEMENT_3D('',#61127,#24929,#24930);
#21262=AXIS2_PLACEMENT_3D('',#61128,#24931,#24932);
#21263=AXIS2_PLACEMENT_3D('',#61131,#24933,#24934);
#21264=AXIS2_PLACEMENT_3D('',#61133,#24935,#24936);
#21265=AXIS2_PLACEMENT_3D('',#61134,#24937,#24938);
#21266=AXIS2_PLACEMENT_3D('',#61135,#24939,#24940);
#21267=AXIS2_PLACEMENT_3D('',#61138,#24941,#24942);
#21268=AXIS2_PLACEMENT_3D('',#61140,#24943,#24944);
#21269=AXIS2_PLACEMENT_3D('',#61141,#24945,#24946);
#21270=AXIS2_PLACEMENT_3D('',#61142,#24947,#24948);
#21271=AXIS2_PLACEMENT_3D('',#61145,#24949,#24950);
#21272=AXIS2_PLACEMENT_3D('',#61148,#24953,#24954);
#21273=AXIS2_PLACEMENT_3D('',#61151,#24955,#24956);
#21274=AXIS2_PLACEMENT_3D('',#61154,#24959,#24960);
#21275=AXIS2_PLACEMENT_3D('',#61157,#24963,#24964);
#21276=AXIS2_PLACEMENT_3D('',#61160,#24965,#24966);
#21277=AXIS2_PLACEMENT_3D('',#61162,#24967,#24968);
#21278=AXIS2_PLACEMENT_3D('',#61163,#24969,#24970);
#21279=AXIS2_PLACEMENT_3D('',#61164,#24971,#24972);
#21280=AXIS2_PLACEMENT_3D('',#61166,#24973,#24974);
#21281=AXIS2_PLACEMENT_3D('',#61169,#24977,#24978);
#21282=AXIS2_PLACEMENT_3D('',#61174,#24981,#24982);
#21283=AXIS2_PLACEMENT_3D('',#61175,#24983,#24984);
#21284=AXIS2_PLACEMENT_3D('',#61180,#24987,#24988);
#21285=AXIS2_PLACEMENT_3D('',#61181,#24989,#24990);
#21286=AXIS2_PLACEMENT_3D('',#61184,#24991,#24992);
#21287=AXIS2_PLACEMENT_3D('',#61186,#24993,#24994);
#21288=AXIS2_PLACEMENT_3D('',#61187,#24995,#24996);
#21289=AXIS2_PLACEMENT_3D('',#61188,#24997,#24998);
#21290=AXIS2_PLACEMENT_3D('',#61191,#25001,#25002);
#21291=AXIS2_PLACEMENT_3D('',#61194,#25003,#25004);
#21292=AXIS2_PLACEMENT_3D('',#61197,#25007,#25008);
#21293=AXIS2_PLACEMENT_3D('',#61200,#25009,#25010);
#21294=AXIS2_PLACEMENT_3D('',#61202,#25011,#25012);
#21295=AXIS2_PLACEMENT_3D('',#61203,#25013,#25014);
#21296=AXIS2_PLACEMENT_3D('',#61204,#25015,#25016);
#21297=AXIS2_PLACEMENT_3D('',#61207,#25019,#25020);
#21298=AXIS2_PLACEMENT_3D('',#61210,#25023,#25024);
#21299=AXIS2_PLACEMENT_3D('',#61213,#25025,#25026);
#21300=AXIS2_PLACEMENT_3D('',#61215,#25027,#25028);
#21301=AXIS2_PLACEMENT_3D('',#61216,#25029,#25030);
#21302=AXIS2_PLACEMENT_3D('',#61217,#25031,#25032);
#21303=AXIS2_PLACEMENT_3D('',#61220,#25033,#25034);
#21304=AXIS2_PLACEMENT_3D('',#61222,#25035,#25036);
#21305=AXIS2_PLACEMENT_3D('',#61223,#25037,#25038);
#21306=AXIS2_PLACEMENT_3D('',#61224,#25039,#25040);
#21307=AXIS2_PLACEMENT_3D('',#61227,#25041,#25042);
#21308=AXIS2_PLACEMENT_3D('',#61230,#25045,#25046);
#21309=AXIS2_PLACEMENT_3D('',#61233,#25047,#25048);
#21310=AXIS2_PLACEMENT_3D('',#61235,#25049,#25050);
#21311=AXIS2_PLACEMENT_3D('',#61236,#25051,#25052);
#21312=AXIS2_PLACEMENT_3D('',#61237,#25053,#25054);
#21313=AXIS2_PLACEMENT_3D('',#61240,#25057,#25058);
#21314=AXIS2_PLACEMENT_3D('',#61245,#25061,#25062);
#21315=AXIS2_PLACEMENT_3D('',#61246,#25063,#25064);
#21316=AXIS2_PLACEMENT_3D('',#61249,#25065,#25066);
#21317=AXIS2_PLACEMENT_3D('',#61251,#25067,#25068);
#21318=AXIS2_PLACEMENT_3D('',#61252,#25069,#25070);
#21319=AXIS2_PLACEMENT_3D('',#61253,#25071,#25072);
#21320=AXIS2_PLACEMENT_3D('',#61256,#25075,#25076);
#21321=AXIS2_PLACEMENT_3D('',#61259,#25079,#25080);
#21322=AXIS2_PLACEMENT_3D('',#61262,#25081,#25082);
#21323=AXIS2_PLACEMENT_3D('',#61265,#25085,#25086);
#21324=AXIS2_PLACEMENT_3D('',#61267,#25087,#25088);
#21325=AXIS2_PLACEMENT_3D('',#61268,#25089,#25090);
#21326=AXIS2_PLACEMENT_3D('',#61269,#25091,#25092);
#21327=AXIS2_PLACEMENT_3D('',#61272,#25095,#25096);
#21328=AXIS2_PLACEMENT_3D('',#61274,#25097,#25098);
#21329=AXIS2_PLACEMENT_3D('',#61277,#25101,#25102);
#21330=AXIS2_PLACEMENT_3D('',#61345,#25105,#25106);
#21331=AXIS2_PLACEMENT_3D('',#61346,#25107,#25108);
#21332=AXIS2_PLACEMENT_3D('',#61378,#25109,#25110);
#21333=AXIS2_PLACEMENT_3D('',#61379,#25111,#25112);
#21334=AXIS2_PLACEMENT_3D('',#61386,#25113,#25114);
#21335=AXIS2_PLACEMENT_3D('',#61387,#25115,#25116);
#21336=AXIS2_PLACEMENT_3D('',#61388,#25117,#25118);
#21337=AXIS2_PLACEMENT_3D('',#61390,#25120,#25121);
#21338=AXIS2_PLACEMENT_3D('',#61393,#25123,#25124);
#21339=AXIS2_PLACEMENT_3D('',#61395,#25125,#25126);
#21340=AXIS2_PLACEMENT_3D('',#61396,#25127,#25128);
#21341=AXIS2_PLACEMENT_3D('',#61398,#25130,#25131);
#21342=AXIS2_PLACEMENT_3D('',#61400,#25133,#25134);
#21343=AXIS2_PLACEMENT_3D('',#61401,#25135,#25136);
#21344=AXIS2_PLACEMENT_3D('',#61402,#25137,#25138);
#21345=AXIS2_PLACEMENT_3D('',#61404,#25140,#25141);
#21346=AXIS2_PLACEMENT_3D('',#61408,#25143,#25144);
#21347=AXIS2_PLACEMENT_3D('',#61410,#25146,#25147);
#21348=AXIS2_PLACEMENT_3D('',#61413,#25150,#25151);
#21349=AXIS2_PLACEMENT_3D('',#61415,#25153,#25154);
#21350=AXIS2_PLACEMENT_3D('',#61417,#25155,#25156);
#21351=AXIS2_PLACEMENT_3D('',#61419,#25157,#25158);
#21352=AXIS2_PLACEMENT_3D('',#61420,#25159,#25160);
#21353=AXIS2_PLACEMENT_3D('',#61421,#25161,#25162);
#21354=AXIS2_PLACEMENT_3D('',#61423,#25163,#25164);
#21355=AXIS2_PLACEMENT_3D('',#61425,#25166,#25167);
#21356=AXIS2_PLACEMENT_3D('',#61427,#25168,#25169);
#21357=AXIS2_PLACEMENT_3D('',#61429,#25170,#25171);
#21358=AXIS2_PLACEMENT_3D('',#61430,#25172,#25173);
#21359=AXIS2_PLACEMENT_3D('',#61431,#25174,#25175);
#21360=AXIS2_PLACEMENT_3D('',#61433,#25176,#25177);
#21361=AXIS2_PLACEMENT_3D('',#61434,#25178,#25179);
#21362=AXIS2_PLACEMENT_3D('',#61438,#25181,#25182);
#21363=AXIS2_PLACEMENT_3D('',#61439,#25183,#25184);
#21364=AXIS2_PLACEMENT_3D('',#61441,#25185,#25186);
#21365=AXIS2_PLACEMENT_3D('',#61443,#25187,#25188);
#21366=AXIS2_PLACEMENT_3D('',#61445,#25189,#25190);
#21367=AXIS2_PLACEMENT_3D('',#61446,#25191,#25192);
#21368=AXIS2_PLACEMENT_3D('',#61447,#25193,#25194);
#21369=AXIS2_PLACEMENT_3D('',#61449,#25195,#25196);
#21370=AXIS2_PLACEMENT_3D('',#61450,#25197,#25198);
#21371=AXIS2_PLACEMENT_3D('',#61451,#25199,#25200);
#21372=AXIS2_PLACEMENT_3D('',#61453,#25201,#25202);
#21373=AXIS2_PLACEMENT_3D('',#61455,#25203,#25204);
#21374=AXIS2_PLACEMENT_3D('',#61456,#25205,#25206);
#21375=AXIS2_PLACEMENT_3D('',#61457,#25207,#25208);
#21376=AXIS2_PLACEMENT_3D('',#61460,#25210,#25211);
#21377=AXIS2_PLACEMENT_3D('',#61461,#25212,#25213);
#21378=AXIS2_PLACEMENT_3D('',#61463,#25214,#25215);
#21379=AXIS2_PLACEMENT_3D('',#61465,#25216,#25217);
#21380=AXIS2_PLACEMENT_3D('',#61466,#25218,#25219);
#21381=AXIS2_PLACEMENT_3D('',#61467,#25220,#25221);
#21382=AXIS2_PLACEMENT_3D('',#61470,#25223,#25224);
#21383=AXIS2_PLACEMENT_3D('',#61471,#25225,#25226);
#21384=AXIS2_PLACEMENT_3D('',#61476,#25228,#25229);
#21385=AXIS2_PLACEMENT_3D('',#61479,#25231,#25232);
#21386=AXIS2_PLACEMENT_3D('',#61480,#25233,#25234);
#21387=AXIS2_PLACEMENT_3D('',#61498,#25237,#25238);
#21388=AXIS2_PLACEMENT_3D('',#61518,#25241,#25242);
#21389=AXIS2_PLACEMENT_3D('',#61519,#25243,#25244);
#21390=AXIS2_PLACEMENT_3D('',#61520,#25245,#25246);
#21391=AXIS2_PLACEMENT_3D('',#61537,#25247,#25248);
#21392=AXIS2_PLACEMENT_3D('',#61556,#25249,#25250);
#21393=AXIS2_PLACEMENT_3D('',#61562,#25254,#25255);
#21394=AXIS2_PLACEMENT_3D('',#61564,#25256,#25257);
#21395=AXIS2_PLACEMENT_3D('',#61566,#25259,#25260);
#21396=AXIS2_PLACEMENT_3D('',#61569,#25262,#25263);
#21397=AXIS2_PLACEMENT_3D('',#61570,#25264,#25265);
#21398=AXIS2_PLACEMENT_3D('',#61572,#25267,#25268);
#21399=AXIS2_PLACEMENT_3D('',#61574,#25269,#25270);
#21400=AXIS2_PLACEMENT_3D('',#61576,#25271,#25272);
#21401=AXIS2_PLACEMENT_3D('',#61577,#25273,#25274);
#21402=AXIS2_PLACEMENT_3D('',#61578,#25275,#25276);
#21403=AXIS2_PLACEMENT_3D('',#61580,#25277,#25278);
#21404=AXIS2_PLACEMENT_3D('',#61581,#25279,#25280);
#21405=AXIS2_PLACEMENT_3D('',#61583,#25281,#25282);
#21406=AXIS2_PLACEMENT_3D('',#61584,#25283,#25284);
#21407=AXIS2_PLACEMENT_3D('',#61585,#25285,#25286);
#21408=AXIS2_PLACEMENT_3D('',#61587,#25287,#25288);
#21409=AXIS2_PLACEMENT_3D('',#61589,#25289,#25290);
#21410=AXIS2_PLACEMENT_3D('',#61590,#25291,#25292);
#21411=AXIS2_PLACEMENT_3D('',#61591,#25293,#25294);
#21412=AXIS2_PLACEMENT_3D('',#61593,#25295,#25296);
#21413=AXIS2_PLACEMENT_3D('',#61594,#25297,#25298);
#21414=AXIS2_PLACEMENT_3D('',#61596,#25299,#25300);
#21415=AXIS2_PLACEMENT_3D('',#61597,#25301,#25302);
#21416=AXIS2_PLACEMENT_3D('',#61598,#25303,#25304);
#21417=AXIS2_PLACEMENT_3D('',#61600,#25305,#25306);
#21418=AXIS2_PLACEMENT_3D('',#61602,#25307,#25308);
#21419=AXIS2_PLACEMENT_3D('',#61603,#25309,#25310);
#21420=AXIS2_PLACEMENT_3D('',#61604,#25311,#25312);
#21421=AXIS2_PLACEMENT_3D('',#61605,#25313,#25314);
#21422=AXIS2_PLACEMENT_3D('',#61606,#25315,#25316);
#21423=AXIS2_PLACEMENT_3D('',#61607,#25317,#25318);
#21424=AXIS2_PLACEMENT_3D('',#61608,#25319,#25320);
#21425=AXIS2_PLACEMENT_3D('',#61609,#25321,#25322);
#21426=AXIS2_PLACEMENT_3D('',#61610,#25323,#25324);
#21427=AXIS2_PLACEMENT_3D('',#61611,#25325,#25326);
#21428=AXIS2_PLACEMENT_3D('',#61612,#25327,#25328);
#21429=AXIS2_PLACEMENT_3D('',#61614,#25329,#25330);
#21430=AXIS2_PLACEMENT_3D('',#61615,#25331,#25332);
#21431=AXIS2_PLACEMENT_3D('',#61617,#25333,#25334);
#21432=AXIS2_PLACEMENT_3D('',#61620,#25336,#25337);
#21433=AXIS2_PLACEMENT_3D('',#61621,#25338,#25339);
#21434=AXIS2_PLACEMENT_3D('',#61623,#25341,#25342);
#21435=AXIS2_PLACEMENT_3D('',#61624,#25343,#25344);
#21436=AXIS2_PLACEMENT_3D('',#61625,#25345,#25346);
#24929=DIRECTION('axis',(0.,0.,1.));
#24930=DIRECTION('refdir',(1.,0.,0.));
#24931=DIRECTION('center_axis',(0.408248290463864,-0.816496580927723,0.408248290463868));
#24932=DIRECTION('ref_axis',(0.577350269189627,0.577350269189627,0.577350269189623));
#24933=DIRECTION('center_axis',(1.,0.,0.));
#24934=DIRECTION('ref_axis',(0.,0.,1.));
#24935=DIRECTION('center_axis',(0.,1.,0.));
#24936=DIRECTION('ref_axis',(1.,0.,0.));
#24937=DIRECTION('center_axis',(0.,0.,1.));
#24938=DIRECTION('ref_axis',(0.,1.,0.));
#24939=DIRECTION('center_axis',(0.408248290463864,-0.408248290463861,-0.816496580927727));
#24940=DIRECTION('ref_axis',(0.577350269189628,-0.577350269189626,0.577350269189624));
#24941=DIRECTION('center_axis',(0.,-1.,0.));
#24942=DIRECTION('ref_axis',(0.,0.,1.));
#24943=DIRECTION('center_axis',(1.,0.,0.));
#24944=DIRECTION('ref_axis',(0.,-1.,0.));
#24945=DIRECTION('center_axis',(0.,0.,1.));
#24946=DIRECTION('ref_axis',(1.,0.,0.));
#24947=DIRECTION('center_axis',(-1.,0.,0.));
#24948=DIRECTION('ref_axis',(0.,-0.707106781186547,0.707106781186548));
#24949=DIRECTION('center_axis',(1.,0.,1.38777878078144E-15));
#24950=DIRECTION('ref_axis',(-1.38777878078144E-15,0.,1.));
#24951=DIRECTION('',(1.,0.,0.));
#24952=DIRECTION('',(-1.,0.,0.));
#24953=DIRECTION('center_axis',(0.,0.,1.));
#24954=DIRECTION('ref_axis',(0.707106781186548,-0.707106781186547,0.));
#24955=DIRECTION('center_axis',(0.,0.,1.));
#24956=DIRECTION('ref_axis',(0.,-1.,0.));
#24957=DIRECTION('',(0.,0.,1.));
#24958=DIRECTION('',(0.,0.,-1.));
#24959=DIRECTION('center_axis',(0.,1.,0.));
#24960=DIRECTION('ref_axis',(0.707106781186548,0.,0.707106781186548));
#24961=DIRECTION('',(0.,-1.,0.));
#24962=DIRECTION('',(0.,1.,0.));
#24963=DIRECTION('center_axis',(0.408248290463864,-0.816496580927728,-0.408248290463859));
#24964=DIRECTION('ref_axis',(0.577350269189632,0.577350269189623,-0.577350269189623));
#24965=DIRECTION('center_axis',(0.,0.,-1.));
#24966=DIRECTION('ref_axis',(1.,0.,0.));
#24967=DIRECTION('center_axis',(0.,1.,0.));
#24968=DIRECTION('ref_axis',(0.,0.,-1.));
#24969=DIRECTION('center_axis',(1.,0.,0.));
#24970=DIRECTION('ref_axis',(0.,1.,0.));
#24971=DIRECTION('center_axis',(0.,1.,0.));
#24972=DIRECTION('ref_axis',(0.707106781186548,0.,-0.707106781186548));
#24973=DIRECTION('center_axis',(0.,1.,0.));
#24974=DIRECTION('ref_axis',(1.,0.,0.));
#24975=DIRECTION('',(0.,1.,0.));
#24976=DIRECTION('',(0.,-1.,0.));
#24977=DIRECTION('center_axis',(-1.,0.,0.));
#24978=DIRECTION('ref_axis',(0.,0.707106781186548,-0.707106781186548));
#24979=DIRECTION('',(1.,0.,0.));
#24980=DIRECTION('',(-1.,0.,0.));
#24981=DIRECTION('center_axis',(0.707106781186547,-0.707106781186549,0.));
#24982=DIRECTION('ref_axis',(0.707106781186548,0.707106781186546,0.));
#24983=DIRECTION('center_axis',(1.,0.,0.));
#24984=DIRECTION('ref_axis',(0.,0.707106781186548,0.707106781186548));
#24985=DIRECTION('',(1.,0.,0.));
#24986=DIRECTION('',(-1.,0.,0.));
#24987=DIRECTION('center_axis',(0.707106781186546,-0.707106781186549,-1.96261557335471E-15));
#24988=DIRECTION('ref_axis',(-0.707106781186549,-0.707106781186546,-1.9626155733547E-15));
#24989=DIRECTION('center_axis',(-0.408248290463864,-0.408248290463859,-0.816496580927728));
#24990=DIRECTION('ref_axis',(0.577350269189629,0.577350269189627,-0.577350269189622));
#24991=DIRECTION('center_axis',(0.,0.,-1.));
#24992=DIRECTION('ref_axis',(1.,0.,0.));
#24993=DIRECTION('center_axis',(0.,1.,0.));
#24994=DIRECTION('ref_axis',(0.,0.,-1.));
#24995=DIRECTION('center_axis',(1.,0.,-2.77555756156289E-15));
#24996=DIRECTION('ref_axis',(0.,1.,0.));
#24997=DIRECTION('center_axis',(0.,1.,0.));
#24998=DIRECTION('ref_axis',(0.707106781186548,0.,-0.707106781186548));
#24999=DIRECTION('',(0.,1.,0.));
#25000=DIRECTION('',(0.,-1.,0.));
#25001=DIRECTION('center_axis',(-1.,0.,0.));
#25002=DIRECTION('ref_axis',(0.,0.707106781186548,-0.707106781186548));
#25003=DIRECTION('center_axis',(1.,0.,-2.77555756156289E-15));
#25004=DIRECTION('ref_axis',(-2.77555756156289E-15,0.,-1.));
#25005=DIRECTION('',(1.,0.,0.));
#25006=DIRECTION('',(-1.,0.,0.));
#25007=DIRECTION('center_axis',(0.408248290463863,0.408248290463863,-0.816496580927726));
#25008=DIRECTION('ref_axis',(0.577350269189626,0.577350269189624,0.577350269189628));
#25009=DIRECTION('center_axis',(1.,-5.55111512312578E-15,0.));
#25010=DIRECTION('ref_axis',(0.,0.,1.));
#25011=DIRECTION('center_axis',(0.,1.,0.));
#25012=DIRECTION('ref_axis',(1.,0.,0.));
#25013=DIRECTION('center_axis',(0.,0.,1.));
#25014=DIRECTION('ref_axis',(0.,1.,0.));
#25015=DIRECTION('center_axis',(0.,1.,0.));
#25016=DIRECTION('ref_axis',(0.707106781186548,0.,0.707106781186548));
#25017=DIRECTION('',(0.,1.,0.));
#25018=DIRECTION('',(0.,-1.,0.));
#25019=DIRECTION('center_axis',(0.,0.,-1.));
#25020=DIRECTION('ref_axis',(0.707106781186548,0.707106781186548,0.));
#25021=DIRECTION('',(0.,0.,1.));
#25022=DIRECTION('',(0.,0.,-1.));
#25023=DIRECTION('center_axis',(-0.408248290463864,0.408248290463859,-0.816496580927728));
#25024=DIRECTION('ref_axis',(-0.577350269189629,0.577350269189627,0.577350269189622));
#25025=DIRECTION('center_axis',(0.,0.,1.));
#25026=DIRECTION('ref_axis',(-1.,0.,0.));
#25027=DIRECTION('center_axis',(0.,1.,0.));
#25028=DIRECTION('ref_axis',(0.,0.,1.));
#25029=DIRECTION('center_axis',(-1.,0.,2.77555756156289E-15));
#25030=DIRECTION('ref_axis',(0.,1.,0.));
#25031=DIRECTION('center_axis',(0.408248290463864,-0.816496580927728,-0.408248290463859));
#25032=DIRECTION('ref_axis',(-0.577350269189631,-0.577350269189624,0.577350269189622));
#25033=DIRECTION('center_axis',(0.,0.,1.));
#25034=DIRECTION('ref_axis',(0.,-1.,0.));
#25035=DIRECTION('center_axis',(-1.,0.,0.));
#25036=DIRECTION('ref_axis',(0.,0.,1.));
#25037=DIRECTION('center_axis',(0.,-1.,0.));
#25038=DIRECTION('ref_axis',(-1.,0.,0.));
#25039=DIRECTION('center_axis',(-1.,0.,0.));
#25040=DIRECTION('ref_axis',(0.,-0.707106781186547,0.707106781186548));
#25041=DIRECTION('center_axis',(-1.,0.,0.));
#25042=DIRECTION('ref_axis',(0.,-1.,0.));
#25043=DIRECTION('',(-1.,0.,0.));
#25044=DIRECTION('',(1.,0.,0.));
#25045=DIRECTION('center_axis',(-0.408248290463864,-0.816496580927728,0.408248290463859));
#25046=DIRECTION('ref_axis',(-0.577350269189632,0.577350269189623,0.577350269189623));
#25047=DIRECTION('center_axis',(0.,0.,1.));
#25048=DIRECTION('ref_axis',(-1.,0.,0.));
#25049=DIRECTION('center_axis',(0.,1.,0.));
#25050=DIRECTION('ref_axis',(0.,0.,1.));
#25051=DIRECTION('center_axis',(-1.,0.,0.));
#25052=DIRECTION('ref_axis',(0.,1.,0.));
#25053=DIRECTION('center_axis',(0.,1.,0.));
#25054=DIRECTION('ref_axis',(-0.707106781186548,0.,0.707106781186548));
#25055=DIRECTION('',(0.,-1.,0.));
#25056=DIRECTION('',(0.,1.,0.));
#25057=DIRECTION('center_axis',(1.,0.,0.));
#25058=DIRECTION('ref_axis',(0.,0.707106781186548,0.707106781186548));
#25059=DIRECTION('',(-1.,0.,0.));
#25060=DIRECTION('',(1.,0.,0.));
#25061=DIRECTION('center_axis',(-0.707106781186547,-0.707106781186549,0.));
#25062=DIRECTION('ref_axis',(-0.707106781186548,0.707106781186546,0.));
#25063=DIRECTION('center_axis',(-0.408248290463864,-0.816496580927723,-0.408248290463868));
#25064=DIRECTION('ref_axis',(-0.577350269189623,0.577350269189632,-0.577350269189623));
#25065=DIRECTION('center_axis',(0.,0.,-1.));
#25066=DIRECTION('ref_axis',(-1.,0.,0.));
#25067=DIRECTION('center_axis',(-1.,0.,0.));
#25068=DIRECTION('ref_axis',(0.,0.707106781186548,-0.707106781186548));
#25069=DIRECTION('center_axis',(0.,1.,0.));
#25070=DIRECTION('ref_axis',(-0.707106781186549,0.,-0.707106781186546));
#25071=DIRECTION('center_axis',(0.,0.,1.));
#25072=DIRECTION('ref_axis',(-0.707106781186548,0.707106781186548,0.));
#25073=DIRECTION('',(0.,0.,1.));
#25074=DIRECTION('',(0.,0.,-1.));
#25075=DIRECTION('center_axis',(0.,1.,0.));
#25076=DIRECTION('ref_axis',(-0.707106781186548,0.,0.707106781186548));
#25077=DIRECTION('',(0.,1.,0.));
#25078=DIRECTION('',(0.,-1.,0.));
#25079=DIRECTION('center_axis',(0.,0.,-1.));
#25080=DIRECTION('ref_axis',(-0.707106781186548,-0.707106781186547,0.));
#25081=DIRECTION('center_axis',(0.,0.,1.));
#25082=DIRECTION('ref_axis',(-1.,0.,0.));
#25083=DIRECTION('',(0.,0.,1.));
#25084=DIRECTION('',(0.,0.,-1.));
#25085=DIRECTION('center_axis',(0.408248290463864,-0.816496580927723,0.408248290463868));
#25086=DIRECTION('ref_axis',(-0.577350269189621,-0.577350269189627,-0.57735026918963));
#25087=DIRECTION('center_axis',(0.,-1.,0.));
#25088=DIRECTION('ref_axis',(-0.707106781186549,0.,-0.707106781186546));
#25089=DIRECTION('center_axis',(-1.,0.,0.));
#25090=DIRECTION('ref_axis',(0.,-0.707106781186546,-0.707106781186549));
#25091=DIRECTION('center_axis',(1.,0.,0.));
#25092=DIRECTION('ref_axis',(0.,0.707106781186548,0.707106781186548));
#25093=DIRECTION('',(-1.,0.,0.));
#25094=DIRECTION('',(1.,0.,0.));
#25095=DIRECTION('center_axis',(0.,0.,1.));
#25096=DIRECTION('ref_axis',(-0.707106781186548,0.707106781186548,0.));
#25097=DIRECTION('center_axis',(0.,0.,1.));
#25098=DIRECTION('ref_axis',(0.,1.,0.));
#25099=DIRECTION('',(0.,0.,1.));
#25100=DIRECTION('',(0.,0.,-1.));
#25101=DIRECTION('center_axis',(0.,0.,-1.));
#25102=DIRECTION('ref_axis',(0.707106781186548,0.707106781186548,0.));
#25103=DIRECTION('',(0.,0.,1.));
#25104=DIRECTION('',(0.,0.,-1.));
#25105=DIRECTION('center_axis',(0.408248290463864,-0.408248290463859,-0.816496580927728));
#25106=DIRECTION('ref_axis',(-0.57735026918963,0.577350269189624,-0.577350269189624));
#25107=DIRECTION('center_axis',(0.,1.,0.));
#25108=DIRECTION('ref_axis',(-0.707106781186549,0.,-0.707106781186546));
#25109=DIRECTION('center_axis',(0.,0.,-1.));
#25110=DIRECTION('ref_axis',(1.,0.,0.));
#25111=DIRECTION('center_axis',(0.,0.,-1.));
#25112=DIRECTION('ref_axis',(1.,0.,0.));
#25113=DIRECTION('center_axis',(-0.408248290463864,-0.816496580927727,0.40824829046386));
#25114=DIRECTION('ref_axis',(0.577350269189628,-0.577350269189625,-0.577350269189624));
#25115=DIRECTION('center_axis',(1.,0.,0.));
#25116=DIRECTION('ref_axis',(0.,-0.707106781186546,-0.707106781186549));
#25117=DIRECTION('center_axis',(1.,0.,0.));
#25118=DIRECTION('ref_axis',(0.,0.,-1.));
#25119=DIRECTION('',(0.,0.,1.));
#25120=DIRECTION('center_axis',(0.,1.,0.));
#25121=DIRECTION('ref_axis',(1.,0.,0.));
#25122=DIRECTION('',(-1.,0.,0.));
#25123=DIRECTION('center_axis',(0.,-1.,0.));
#25124=DIRECTION('ref_axis',(1.,0.,0.));
#25125=DIRECTION('center_axis',(0.,-1.,0.));
#25126=DIRECTION('ref_axis',(1.,0.,0.));
#25127=DIRECTION('center_axis',(-1.,0.,0.));
#25128=DIRECTION('ref_axis',(0.,0.,1.));
#25129=DIRECTION('',(0.,1.,0.));
#25130=DIRECTION('center_axis',(0.,1.,0.));
#25131=DIRECTION('ref_axis',(-0.707106781186548,0.,-0.707106781186548));
#25132=DIRECTION('',(0.,-1.,0.));
#25133=DIRECTION('center_axis',(1.,0.,0.));
#25134=DIRECTION('ref_axis',(0.,0.,-1.));
#25135=DIRECTION('center_axis',(0.,1.,0.));
#25136=DIRECTION('ref_axis',(0.,0.,1.));
#25137=DIRECTION('center_axis',(1.,0.,0.));
#25138=DIRECTION('ref_axis',(0.,-0.707106781186547,-0.707106781186548));
#25139=DIRECTION('',(1.,0.,0.));
#25140=DIRECTION('center_axis',(-1.,0.,0.));
#25141=DIRECTION('ref_axis',(0.,0.707106781186548,-0.707106781186548));
#25142=DIRECTION('',(1.,0.,0.));
#25143=DIRECTION('center_axis',(-0.707106781186546,-0.707106781186549,1.96261557335471E-15));
#25144=DIRECTION('ref_axis',(0.707106781186549,-0.707106781186546,1.9626155733547E-15));
#25145=DIRECTION('',(-1.,0.,0.));
#25146=DIRECTION('center_axis',(0.,1.,0.));
#25147=DIRECTION('ref_axis',(-0.707106781186548,0.,-0.707106781186548));
#25148=DIRECTION('',(0.,-1.,0.));
#25149=DIRECTION('',(0.,1.,0.));
#25150=DIRECTION('center_axis',(0.,1.,0.));
#25151=DIRECTION('ref_axis',(0.,0.,1.));
#25152=DIRECTION('',(0.,0.,-1.));
#25153=DIRECTION('center_axis',(0.,0.,1.));
#25154=DIRECTION('ref_axis',(1.,0.,0.));
#25155=DIRECTION('center_axis',(0.,0.,-1.));
#25156=DIRECTION('ref_axis',(1.,0.,0.));
#25157=DIRECTION('center_axis',(0.,-1.,0.));
#25158=DIRECTION('ref_axis',(-1.,0.,0.));
#25159=DIRECTION('center_axis',(0.,0.,1.));
#25160=DIRECTION('ref_axis',(1.,0.,0.));
#25161=DIRECTION('center_axis',(0.,0.,1.));
#25162=DIRECTION('ref_axis',(1.,0.,0.));
#25163=DIRECTION('center_axis',(0.,0.,1.));
#25164=DIRECTION('ref_axis',(1.,0.,0.));
#25165=DIRECTION('',(0.,0.,1.));
#25166=DIRECTION('center_axis',(0.,0.,1.));
#25167=DIRECTION('ref_axis',(1.,0.,0.));
#25168=DIRECTION('center_axis',(0.,0.,-1.));
#25169=DIRECTION('ref_axis',(1.,0.,0.));
#25170=DIRECTION('center_axis',(1.81408990951823E-16,-1.,0.));
#25171=DIRECTION('ref_axis',(-1.,-1.81408990951823E-16,0.));
#25172=DIRECTION('center_axis',(0.,0.,1.));
#25173=DIRECTION('ref_axis',(1.,0.,0.));
#25174=DIRECTION('center_axis',(0.,0.,1.));
#25175=DIRECTION('ref_axis',(1.,0.,0.));
#25176=DIRECTION('center_axis',(0.,0.,1.));
#25177=DIRECTION('ref_axis',(-1.,0.,0.));
#25178=DIRECTION('center_axis',(0.,0.,1.));
#25179=DIRECTION('ref_axis',(1.,0.,0.));
#25180=DIRECTION('',(0.,0.,-1.));
#25181=DIRECTION('center_axis',(0.,0.,-1.));
#25182=DIRECTION('ref_axis',(1.,0.,0.));
#25183=DIRECTION('center_axis',(0.,0.,-1.));
#25184=DIRECTION('ref_axis',(1.,0.,0.));
#25185=DIRECTION('center_axis',(0.,0.,-1.));
#25186=DIRECTION('ref_axis',(1.,0.,0.));
#25187=DIRECTION('center_axis',(0.,0.,-1.));
#25188=DIRECTION('ref_axis',(1.,0.,0.));
#25189=DIRECTION('center_axis',(0.,0.,-1.));
#25190=DIRECTION('ref_axis',(1.,0.,0.));
#25191=DIRECTION('center_axis',(0.,0.,-1.));
#25192=DIRECTION('ref_axis',(1.,0.,0.));
#25193=DIRECTION('center_axis',(0.,0.,1.));
#25194=DIRECTION('ref_axis',(-1.,0.,0.));
#25195=DIRECTION('center_axis',(0.,0.,-1.));
#25196=DIRECTION('ref_axis',(1.,0.,0.));
#25197=DIRECTION('center_axis',(-1.82088236683647E-16,1.,0.));
#25198=DIRECTION('ref_axis',(1.,1.82088236683647E-16,0.));
#25199=DIRECTION('center_axis',(0.,1.,0.));
#25200=DIRECTION('ref_axis',(0.,0.,1.));
#25201=DIRECTION('center_axis',(-1.,0.,0.));
#25202=DIRECTION('ref_axis',(0.,0.,-1.));
#25203=DIRECTION('center_axis',(0.,1.,0.));
#25204=DIRECTION('ref_axis',(1.,0.,0.));
#25205=DIRECTION('center_axis',(0.,1.,0.));
#25206=DIRECTION('ref_axis',(1.,0.,0.));
#25207=DIRECTION('center_axis',(0.,1.,0.));
#25208=DIRECTION('ref_axis',(1.,0.,0.));
#25209=DIRECTION('',(0.,1.,0.));
#25210=DIRECTION('center_axis',(0.,1.,0.));
#25211=DIRECTION('ref_axis',(1.,0.,0.));
#25212=DIRECTION('center_axis',(0.,1.,0.));
#25213=DIRECTION('ref_axis',(0.,0.,1.));
#25214=DIRECTION('center_axis',(-1.,0.,0.));
#25215=DIRECTION('ref_axis',(0.,0.,-1.));
#25216=DIRECTION('center_axis',(0.,1.,0.));
#25217=DIRECTION('ref_axis',(1.,0.,0.));
#25218=DIRECTION('center_axis',(0.,1.,0.));
#25219=DIRECTION('ref_axis',(1.,0.,0.));
#25220=DIRECTION('center_axis',(0.,1.,0.));
#25221=DIRECTION('ref_axis',(1.,0.,0.));
#25222=DIRECTION('',(0.,1.,0.));
#25223=DIRECTION('center_axis',(0.,1.,0.));
#25224=DIRECTION('ref_axis',(1.,0.,0.));
#25225=DIRECTION('center_axis',(0.,-1.,0.));
#25226=DIRECTION('ref_axis',(0.921659373087477,0.,0.387999999999999));
#25227=DIRECTION('',(0.,-1.,0.));
#25228=DIRECTION('center_axis',(-0.707106781186547,0.707106781186548,9.8130778667736E-16));
#25229=DIRECTION('ref_axis',(0.707106781186548,0.707106781186547,-9.81307786677362E-16));
#25230=DIRECTION('',(0.,1.,0.));
#25231=DIRECTION('center_axis',(-0.707106781186548,-0.707106781186547,5.88784672006415E-15));
#25232=DIRECTION('ref_axis',(-0.707106781186547,0.707106781186548,5.88784672006415E-15));
#25233=DIRECTION('center_axis',(1.,0.,0.));
#25234=DIRECTION('ref_axis',(0.,0.921659373087477,0.387999999999999));
#25235=DIRECTION('',(-1.,0.,0.));
#25236=DIRECTION('',(1.,0.,0.));
#25237=DIRECTION('center_axis',(-1.,0.,0.));
#25238=DIRECTION('ref_axis',(0.,-0.921659373087476,0.388));
#25239=DIRECTION('',(-1.,0.,0.));
#25240=DIRECTION('',(1.,0.,0.));
#25241=DIRECTION('center_axis',(1.08557947792634E-16,-4.02936130515309E-16,
-1.));
#25242=DIRECTION('ref_axis',(-0.97786928031163,-0.209216802917009,0.));
#25243=DIRECTION('center_axis',(0.,0.,1.));
#25244=DIRECTION('ref_axis',(1.,0.,0.));
#25245=DIRECTION('center_axis',(-2.11382759593089E-16,-7.1112105974302E-16,
1.));
#25246=DIRECTION('ref_axis',(0.965794610306648,-0.259308254212299,0.));
#25247=DIRECTION('center_axis',(0.,0.,1.));
#25248=DIRECTION('ref_axis',(1.,0.,0.));
#25249=DIRECTION('center_axis',(0.,0.,1.));
#25250=DIRECTION('ref_axis',(1.,0.,0.));
#25251=DIRECTION('',(-1.,0.,0.));
#25252=DIRECTION('',(0.,1.,0.));
#25253=DIRECTION('',(1.,0.,0.));
#25254=DIRECTION('center_axis',(1.,0.,0.));
#25255=DIRECTION('ref_axis',(0.,0.921659373087477,0.387999999999999));
#25256=DIRECTION('center_axis',(-0.707106781186548,-0.707106781186547,1.96261557335472E-15));
#25257=DIRECTION('ref_axis',(-0.707106781186547,0.707106781186548,-1.96261557335472E-15));
#25258=DIRECTION('',(-1.,0.,0.));
#25259=DIRECTION('center_axis',(-1.,0.,0.));
#25260=DIRECTION('ref_axis',(0.,-0.921659373087476,0.388));
#25261=DIRECTION('',(1.,0.,0.));
#25262=DIRECTION('center_axis',(-0.707106781186546,0.707106781186549,0.));
#25263=DIRECTION('ref_axis',(0.707106781186549,0.707106781186546,0.));
#25264=DIRECTION('center_axis',(0.,1.,0.));
#25265=DIRECTION('ref_axis',(-0.921659373087477,0.,0.387999999999999));
#25266=DIRECTION('',(0.,-1.,0.));
#25267=DIRECTION('center_axis',(0.,0.,1.));
#25268=DIRECTION('ref_axis',(-1.,0.,0.));
#25269=DIRECTION('center_axis',(0.,0.,-1.));
#25270=DIRECTION('ref_axis',(1.,0.,0.));
#25271=DIRECTION('center_axis',(0.,1.,0.));
#25272=DIRECTION('ref_axis',(1.,0.,0.));
#25273=DIRECTION('center_axis',(0.,0.,1.));
#25274=DIRECTION('ref_axis',(-1.,0.,0.));
#25275=DIRECTION('center_axis',(0.,0.,1.));
#25276=DIRECTION('ref_axis',(1.,0.,0.));
#25277=DIRECTION('center_axis',(0.,0.,1.));
#25278=DIRECTION('ref_axis',(-1.,0.,0.));
#25279=DIRECTION('center_axis',(0.,0.,1.));
#25280=DIRECTION('ref_axis',(-1.,0.,0.));
#25281=DIRECTION('center_axis',(0.,0.,-1.));
#25282=DIRECTION('ref_axis',(1.,0.,0.));
#25283=DIRECTION('center_axis',(0.,1.,0.));
#25284=DIRECTION('ref_axis',(1.,0.,0.));
#25285=DIRECTION('center_axis',(0.,0.,1.));
#25286=DIRECTION('ref_axis',(-1.,0.,0.));
#25287=DIRECTION('center_axis',(0.,0.,-1.));
#25288=DIRECTION('ref_axis',(1.,0.,0.));
#25289=DIRECTION('center_axis',(0.,1.,0.));
#25290=DIRECTION('ref_axis',(1.,0.,0.));
#25291=DIRECTION('center_axis',(0.,0.,1.));
#25292=DIRECTION('ref_axis',(-1.,0.,0.));
#25293=DIRECTION('center_axis',(0.,0.,1.));
#25294=DIRECTION('ref_axis',(1.,0.,0.));
#25295=DIRECTION('center_axis',(0.,0.,1.));
#25296=DIRECTION('ref_axis',(-1.,0.,0.));
#25297=DIRECTION('center_axis',(0.,0.,1.));
#25298=DIRECTION('ref_axis',(-1.,0.,0.));
#25299=DIRECTION('center_axis',(0.,0.,-1.));
#25300=DIRECTION('ref_axis',(1.,0.,0.));
#25301=DIRECTION('center_axis',(0.,1.,0.));
#25302=DIRECTION('ref_axis',(1.,0.,0.));
#25303=DIRECTION('center_axis',(0.,0.,-1.));
#25304=DIRECTION('ref_axis',(-1.,0.,0.));
#25305=DIRECTION('center_axis',(0.,0.,1.));
#25306=DIRECTION('ref_axis',(1.,0.,0.));
#25307=DIRECTION('center_axis',(0.,-1.,0.));
#25308=DIRECTION('ref_axis',(1.,0.,0.));
#25309=DIRECTION('center_axis',(0.,0.,-1.));
#25310=DIRECTION('ref_axis',(1.,0.,0.));
#25311=DIRECTION('center_axis',(0.,0.,1.));
#25312=DIRECTION('ref_axis',(1.,0.,0.));
#25313=DIRECTION('center_axis',(0.,0.,1.));
#25314=DIRECTION('ref_axis',(1.,0.,0.));
#25315=DIRECTION('center_axis',(0.,0.,1.));
#25316=DIRECTION('ref_axis',(1.,0.,0.));
#25317=DIRECTION('center_axis',(0.,0.,1.));
#25318=DIRECTION('ref_axis',(1.,0.,0.));
#25319=DIRECTION('center_axis',(0.,0.,1.));
#25320=DIRECTION('ref_axis',(1.,0.,0.));
#25321=DIRECTION('center_axis',(0.,1.,0.));
#25322=DIRECTION('ref_axis',(1.,0.,0.));
#25323=DIRECTION('center_axis',(0.,1.,0.));
#25324=DIRECTION('ref_axis',(1.,0.,0.));
#25325=DIRECTION('center_axis',(0.,0.,1.));
#25326=DIRECTION('ref_axis',(1.,0.,0.));
#25327=DIRECTION('center_axis',(0.,0.,1.));
#25328=DIRECTION('ref_axis',(1.,0.,0.));
#25329=DIRECTION('center_axis',(0.,0.,1.));
#25330=DIRECTION('ref_axis',(1.,0.,0.));
#25331=DIRECTION('center_axis',(0.,0.,-1.));
#25332=DIRECTION('ref_axis',(1.,0.,0.));
#25333=DIRECTION('center_axis',(0.,0.,1.));
#25334=DIRECTION('ref_axis',(1.,0.,0.));
#25335=DIRECTION('',(-0.707106781186547,8.65956056235493E-17,-0.707106781186548));
#25336=DIRECTION('center_axis',(0.,0.,-1.));
#25337=DIRECTION('ref_axis',(1.,0.,0.));
#25338=DIRECTION('center_axis',(0.,0.,1.));
#25339=DIRECTION('ref_axis',(1.,0.,0.));
#25340=DIRECTION('',(0.,0.,1.));
#25341=DIRECTION('center_axis',(0.,0.,-1.));
#25342=DIRECTION('ref_axis',(-1.,0.,0.));
#25343=DIRECTION('center_axis',(-1.,0.,0.));
#25344=DIRECTION('ref_axis',(0.,0.,1.));
#25345=DIRECTION('center_axis',(0.,1.,0.));
#25346=DIRECTION('ref_axis',(0.,0.,1.));
#61127=CARTESIAN_POINT('',(0.,0.,0.));
#61128=CARTESIAN_POINT('Origin',(16.744,21.232,44.896));
#61129=CARTESIAN_POINT('',(16.744,21.232,45.696));
#61130=CARTESIAN_POINT('',(16.744,22.032,44.896));
#61131=CARTESIAN_POINT('Origin',(16.744,21.232,44.896));
#61132=CARTESIAN_POINT('',(17.544,21.232,44.896));
#61133=CARTESIAN_POINT('Origin',(16.744,21.232,44.896));
#61134=CARTESIAN_POINT('Origin',(16.744,21.232,44.896));
#61135=CARTESIAN_POINT('Origin',(16.744,3.248,44.896));
#61136=CARTESIAN_POINT('',(16.744,3.248,45.696));
#61137=CARTESIAN_POINT('',(17.544,3.248,44.896));
#61138=CARTESIAN_POINT('Origin',(16.744,3.248,44.896));
#61139=CARTESIAN_POINT('',(16.744,2.448,44.896));
#61140=CARTESIAN_POINT('Origin',(16.744,3.248,44.896));
#61141=CARTESIAN_POINT('Origin',(16.744,3.248,44.896));
#61142=CARTESIAN_POINT('Origin',(-8.772,3.248,44.896));
#61143=CARTESIAN_POINT('',(4.35247056279534,3.248,45.696));
#61144=CARTESIAN_POINT('',(4.35247056279534,2.448,44.896));
#61145=CARTESIAN_POINT('Origin',(4.35247056279534,3.248,44.896));
#61146=CARTESIAN_POINT('',(-8.772,2.448,44.896));
#61147=CARTESIAN_POINT('',(-8.772,3.248,45.696));
#61148=CARTESIAN_POINT('Origin',(16.744,3.248,44.064));
#61149=CARTESIAN_POINT('',(16.744,2.448,39.968));
#61150=CARTESIAN_POINT('',(17.544,3.248,39.968));
#61151=CARTESIAN_POINT('Origin',(16.744,3.248,39.968));
#61152=CARTESIAN_POINT('',(17.544,3.248,44.064));
#61153=CARTESIAN_POINT('',(16.744,2.448,44.064));
#61154=CARTESIAN_POINT('Origin',(16.744,2.448,44.896));
#61155=CARTESIAN_POINT('',(16.744,2.448,45.696));
#61156=CARTESIAN_POINT('',(17.544,2.448,44.896));
#61157=CARTESIAN_POINT('Origin',(16.744,21.232,39.968));
#61158=CARTESIAN_POINT('',(17.544,21.232,39.968));
#61159=CARTESIAN_POINT('',(16.744,22.032,39.968));
#61160=CARTESIAN_POINT('Origin',(16.744,21.232,39.968));
#61161=CARTESIAN_POINT('',(16.744,21.232,39.168));
#61162=CARTESIAN_POINT('Origin',(16.744,21.232,39.968));
#61163=CARTESIAN_POINT('Origin',(16.744,21.232,39.968));
#61164=CARTESIAN_POINT('Origin',(16.744,2.448,39.968));
#61165=CARTESIAN_POINT('',(16.744,3.248,39.168));
#61166=CARTESIAN_POINT('Origin',(16.744,3.248,39.968));
#61167=CARTESIAN_POINT('',(16.744,2.448,39.168));
#61168=CARTESIAN_POINT('',(17.544,2.448,39.968));
#61169=CARTESIAN_POINT('Origin',(8.772,21.232,39.968));
#61170=CARTESIAN_POINT('',(13.056,22.032,39.968));
#61171=CARTESIAN_POINT('',(8.772,22.032,39.968));
#61172=CARTESIAN_POINT('',(12.256,21.232,39.168));
#61173=CARTESIAN_POINT('',(8.772,21.232,39.168));
#61174=CARTESIAN_POINT('Origin',(12.256,21.232,39.968));
#61175=CARTESIAN_POINT('Origin',(-8.772,21.232,44.896));
#61176=CARTESIAN_POINT('',(12.256,21.232,45.696));
#61177=CARTESIAN_POINT('',(-8.772,21.232,45.696));
#61178=CARTESIAN_POINT('',(13.056,22.032,44.896));
#61179=CARTESIAN_POINT('',(-8.772,22.032,44.896));
#61180=CARTESIAN_POINT('Origin',(12.256,21.232,44.896));
#61181=CARTESIAN_POINT('Origin',(12.256,29.392,39.968));
#61182=CARTESIAN_POINT('',(13.056,29.392,39.968));
#61183=CARTESIAN_POINT('',(12.256,30.192,39.968));
#61184=CARTESIAN_POINT('Origin',(12.256,29.392,39.968));
#61185=CARTESIAN_POINT('',(12.256,29.392,39.168));
#61186=CARTESIAN_POINT('Origin',(12.256,29.392,39.968));
#61187=CARTESIAN_POINT('Origin',(12.256,29.392,39.968));
#61188=CARTESIAN_POINT('Origin',(12.256,12.24,39.968));
#61189=CARTESIAN_POINT('',(12.256,12.24,39.168));
#61190=CARTESIAN_POINT('',(13.056,12.24,39.968));
#61191=CARTESIAN_POINT('Origin',(8.772,29.392,39.968));
#61192=CARTESIAN_POINT('',(-12.256,29.392,39.168));
#61193=CARTESIAN_POINT('',(-12.256,30.192,39.968));
#61194=CARTESIAN_POINT('Origin',(-12.256,29.392,39.968));
#61195=CARTESIAN_POINT('',(8.772,30.192,39.968));
#61196=CARTESIAN_POINT('',(8.772,29.392,39.168));
#61197=CARTESIAN_POINT('Origin',(12.256,29.392,44.896));
#61198=CARTESIAN_POINT('',(12.256,29.392,45.696));
#61199=CARTESIAN_POINT('',(12.256,30.192,44.896));
#61200=CARTESIAN_POINT('Origin',(12.256,29.392,44.896));
#61201=CARTESIAN_POINT('',(13.056,29.392,44.896));
#61202=CARTESIAN_POINT('Origin',(12.256,29.392,44.896));
#61203=CARTESIAN_POINT('Origin',(12.256,29.392,44.896));
#61204=CARTESIAN_POINT('Origin',(12.256,12.24,44.896));
#61205=CARTESIAN_POINT('',(13.056,12.24,44.896));
#61206=CARTESIAN_POINT('',(12.256,12.24,45.696));
#61207=CARTESIAN_POINT('Origin',(12.256,29.392,44.064));
#61208=CARTESIAN_POINT('',(12.256,30.192,44.064));
#61209=CARTESIAN_POINT('',(13.056,29.392,44.064));
#61210=CARTESIAN_POINT('Origin',(-12.256,29.392,44.896));
#61211=CARTESIAN_POINT('',(-13.056,29.392,44.896));
#61212=CARTESIAN_POINT('',(-12.256,30.192,44.896));
#61213=CARTESIAN_POINT('Origin',(-12.256,29.392,44.896));
#61214=CARTESIAN_POINT('',(-12.256,29.392,45.696));
#61215=CARTESIAN_POINT('Origin',(-12.256,29.392,44.896));
#61216=CARTESIAN_POINT('Origin',(-12.256,29.392,44.896));
#61217=CARTESIAN_POINT('Origin',(-16.744,3.248,44.896));
#61218=CARTESIAN_POINT('',(-16.744,2.448,44.896));
#61219=CARTESIAN_POINT('',(-17.544,3.248,44.896));
#61220=CARTESIAN_POINT('Origin',(-16.744,3.248,44.896));
#61221=CARTESIAN_POINT('',(-16.744,3.248,45.696));
#61222=CARTESIAN_POINT('Origin',(-16.744,3.248,44.896));
#61223=CARTESIAN_POINT('Origin',(-16.744,3.248,44.896));
#61224=CARTESIAN_POINT('Origin',(-8.772,3.248,44.896));
#61225=CARTESIAN_POINT('',(-4.35247056279534,2.448,44.896));
#61226=CARTESIAN_POINT('',(-4.35247056279534,3.248,45.696));
#61227=CARTESIAN_POINT('Origin',(-4.35247056279534,3.248,44.896));
#61228=CARTESIAN_POINT('',(-8.772,3.248,45.696));
#61229=CARTESIAN_POINT('',(-8.772,2.448,44.896));
#61230=CARTESIAN_POINT('Origin',(-16.744,21.232,44.896));
#61231=CARTESIAN_POINT('',(-17.544,21.232,44.896));
#61232=CARTESIAN_POINT('',(-16.744,22.032,44.896));
#61233=CARTESIAN_POINT('Origin',(-16.744,21.232,44.896));
#61234=CARTESIAN_POINT('',(-16.744,21.232,45.696));
#61235=CARTESIAN_POINT('Origin',(-16.744,21.232,44.896));
#61236=CARTESIAN_POINT('Origin',(-16.744,21.232,44.896));
#61237=CARTESIAN_POINT('Origin',(-16.744,2.448,44.896));
#61238=CARTESIAN_POINT('',(-17.544,2.448,44.896));
#61239=CARTESIAN_POINT('',(-16.744,2.448,45.696));
#61240=CARTESIAN_POINT('Origin',(-8.772,21.232,44.896));
#61241=CARTESIAN_POINT('',(-13.056,22.032,44.896));
#61242=CARTESIAN_POINT('',(-8.772,22.032,44.896));
#61243=CARTESIAN_POINT('',(-12.256,21.232,45.696));
#61244=CARTESIAN_POINT('',(-8.772,21.232,45.696));
#61245=CARTESIAN_POINT('Origin',(-12.256,21.232,44.896));
#61246=CARTESIAN_POINT('Origin',(-16.744,21.232,39.968));
#61247=CARTESIAN_POINT('',(-17.544,21.232,39.968));
#61248=CARTESIAN_POINT('',(-16.744,22.032,39.968));
#61249=CARTESIAN_POINT('Origin',(-16.744,21.232,39.968));
#61250=CARTESIAN_POINT('',(-16.744,21.232,39.168));
#61251=CARTESIAN_POINT('Origin',(-16.744,21.232,39.968));
#61252=CARTESIAN_POINT('Origin',(-16.744,21.232,39.968));
#61253=CARTESIAN_POINT('Origin',(-16.744,21.232,40.8));
#61254=CARTESIAN_POINT('',(-17.544,21.232,40.8));
#61255=CARTESIAN_POINT('',(-16.744,22.032,40.8));
#61256=CARTESIAN_POINT('Origin',(-12.256,12.24,44.896));
#61257=CARTESIAN_POINT('',(-12.256,12.24,45.696));
#61258=CARTESIAN_POINT('',(-13.056,12.24,44.896));
#61259=CARTESIAN_POINT('Origin',(-16.744,3.248,40.8));
#61260=CARTESIAN_POINT('',(-17.544,3.248,39.968));
#61261=CARTESIAN_POINT('',(-16.744,2.448,39.968));
#61262=CARTESIAN_POINT('Origin',(-16.744,3.248,39.968));
#61263=CARTESIAN_POINT('',(-16.744,2.448,40.8));
#61264=CARTESIAN_POINT('',(-17.544,3.248,40.8));
#61265=CARTESIAN_POINT('Origin',(-16.744,3.248,39.968));
#61266=CARTESIAN_POINT('',(-16.744,3.248,39.168));
#61267=CARTESIAN_POINT('Origin',(-16.744,3.248,39.968));
#61268=CARTESIAN_POINT('Origin',(-16.744,3.248,39.968));
#61269=CARTESIAN_POINT('Origin',(-8.772,29.392,44.896));
#61270=CARTESIAN_POINT('',(-8.772,30.192,44.896));
#61271=CARTESIAN_POINT('',(-8.772,29.392,45.696));
#61272=CARTESIAN_POINT('Origin',(-12.256,29.392,40.8));
#61273=CARTESIAN_POINT('',(-13.056,29.392,39.968));
#61274=CARTESIAN_POINT('Origin',(-12.256,29.392,39.968));
#61275=CARTESIAN_POINT('',(-13.056,29.392,40.8));
#61276=CARTESIAN_POINT('',(-12.256,30.192,40.8));
#61277=CARTESIAN_POINT('Origin',(16.744,21.232,44.064));
#61278=CARTESIAN_POINT('',(16.744,22.032,44.064));
#61279=CARTESIAN_POINT('',(17.544,21.232,44.064));
#61280=CARTESIAN_POINT('Ctrl Pts',(7.4948384107818E-16,2.448,45.696));
#61281=CARTESIAN_POINT('Ctrl Pts',(-0.0042297694102402,2.448,45.6960019265802));
#61282=CARTESIAN_POINT('Ctrl Pts',(-0.00845818449221337,2.44800353095933,
45.6960038547636));
#61283=CARTESIAN_POINT('Ctrl Pts',(-0.926069758734644,2.44858567321808,
45.6964214479009));
#61284=CARTESIAN_POINT('Ctrl Pts',(-2.15780484233224,2.59294255969351,45.6969841667508));
#61285=CARTESIAN_POINT('Ctrl Pts',(-3.5684103856049,2.97124337151832,45.6966752349463));
#61286=CARTESIAN_POINT('Ctrl Pts',(-4.10516581642087,3.15568217900954,45.6962732015741));
#61287=CARTESIAN_POINT('Ctrl Pts',(-4.36651858547018,3.25568165343709,45.6959807918452));
#61288=CARTESIAN_POINT('Ctrl Pts',(7.4948384107818E-16,2.448,45.696));
#61289=CARTESIAN_POINT('Ctrl Pts',(-0.00416276422045042,2.448,45.6958022200772));
#61290=CARTESIAN_POINT('Ctrl Pts',(-0.00836699352100908,2.44798339666368,
45.6956042979429));
#61291=CARTESIAN_POINT('Ctrl Pts',(-0.913504058614908,2.4498415415713,45.6527356961232));
#61292=CARTESIAN_POINT('Ctrl Pts',(-2.13405707884003,2.53374268898235,45.5949753639831));
#61293=CARTESIAN_POINT('Ctrl Pts',(-3.56166897255153,2.79399285615006,45.6268807116574));
#61294=CARTESIAN_POINT('Ctrl Pts',(-4.10497083294057,2.93362393613479,45.6682659881586));
#61295=CARTESIAN_POINT('Ctrl Pts',(-4.36653277992524,3.01450371964943,45.6983471985849));
#61296=CARTESIAN_POINT('Ctrl Pts',(7.4948384107818E-16,2.448,45.696));
#61297=CARTESIAN_POINT('Ctrl Pts',(-0.00407497810370066,2.448,45.6954571286858));
#61298=CARTESIAN_POINT('Ctrl Pts',(-0.00817838886308814,2.44799413269538,
45.6949016819103));
#61299=CARTESIAN_POINT('Ctrl Pts',(-0.893431977013438,2.44860632854555,
45.5767431370729));
#61300=CARTESIAN_POINT('Ctrl Pts',(-2.08821913676147,2.46675784665521,45.4140811184592));
#61301=CARTESIAN_POINT('Ctrl Pts',(-3.534931299702,2.53273348711954,45.3978866963668));
#61302=CARTESIAN_POINT('Ctrl Pts',(-4.09594086592657,2.57158546220149,45.4499925192889));
#61303=CARTESIAN_POINT('Ctrl Pts',(-4.36704474249966,2.59586901950321,45.4983996515835));
#61304=CARTESIAN_POINT('Ctrl Pts',(7.4948384107818E-16,2.448,45.696));
#61305=CARTESIAN_POINT('Ctrl Pts',(-0.00398896174508187,2.448,45.6951045051365));
#61306=CARTESIAN_POINT('Ctrl Pts',(-0.0079872843945144,2.448,45.6942070450307));
#61307=CARTESIAN_POINT('Ctrl Pts',(-0.87369611876912,2.44800000000002,45.5001223087092));
#61308=CARTESIAN_POINT('Ctrl Pts',(-2.03938167211534,2.448,45.2359122100003));
#61309=CARTESIAN_POINT('Ctrl Pts',(-3.49454117469163,2.448,45.0734599399993));
#61310=CARTESIAN_POINT('Ctrl Pts',(-4.07699986556522,2.448,45.0613017312264));
#61311=CARTESIAN_POINT('Ctrl Pts',(-4.36811063334064,2.448,45.0763052280038));
#61312=CARTESIAN_POINT('Ctrl Pts',(7.4948384107818E-16,2.448,45.696));
#61313=CARTESIAN_POINT('Ctrl Pts',(-0.00395271020241197,2.448,45.6949547336815));
#61314=CARTESIAN_POINT('Ctrl Pts',(-0.0079050097320282,2.448,45.6939088542388));
#61315=CARTESIAN_POINT('Ctrl Pts',(-0.865284652416804,2.44800000000002,
45.4674065150327));
#61316=CARTESIAN_POINT('Ctrl Pts',(-2.01851098765155,2.448,45.1596990578109));
#61317=CARTESIAN_POINT('Ctrl Pts',(-3.47727706236774,2.448,44.9347642209047));
#61318=CARTESIAN_POINT('Ctrl Pts',(-4.06894992871341,2.448,44.8952825142091));
#61319=CARTESIAN_POINT('Ctrl Pts',(-4.36856368751371,2.448,44.8960197795982));
#61320=CARTESIAN_POINT('',(0.,2.448,45.696));
#61321=CARTESIAN_POINT('Ctrl Pts',(-4.35247056279534,2.448,44.896));
#61322=CARTESIAN_POINT('Ctrl Pts',(-4.05826044258909,2.448,44.896));
#61323=CARTESIAN_POINT('Ctrl Pts',(-3.47197716194173,2.448,44.9355814405115));
#61324=CARTESIAN_POINT('Ctrl Pts',(-2.01851098765155,2.448,45.1596990578109));
#61325=CARTESIAN_POINT('Ctrl Pts',(-0.865284652416804,2.44800000000002,
45.4674065150327));
#61326=CARTESIAN_POINT('Ctrl Pts',(-0.0079050097320282,2.448,45.6939088542388));
#61327=CARTESIAN_POINT('Ctrl Pts',(-0.00395271020241197,2.448,45.6949547336815));
#61328=CARTESIAN_POINT('Ctrl Pts',(7.4948384107818E-16,2.448,45.696));
#61329=CARTESIAN_POINT('',(-0.0438084974115087,2.44807801344885,45.6958602367687));
#61330=CARTESIAN_POINT('Ctrl Pts',(7.4948384107818E-16,2.448,45.696));
#61331=CARTESIAN_POINT('Ctrl Pts',(-0.0146028459483958,2.448,45.6959524518301));
#61332=CARTESIAN_POINT('Ctrl Pts',(-0.029205702201559,2.4480259973895,45.6959058635638));
#61333=CARTESIAN_POINT('Ctrl Pts',(-0.0438084974115087,2.44807801344885,
45.6958602367687));
#61334=CARTESIAN_POINT('Ctrl Pts',(-0.0438084974115087,2.44807801344885,
45.6958602367687));
#61335=CARTESIAN_POINT('Ctrl Pts',(-0.215221081627298,2.44868859567132,
45.6953246539055));
#61336=CARTESIAN_POINT('Ctrl Pts',(-0.572631506599956,2.45743734647924,
45.6944841070415));
#61337=CARTESIAN_POINT('Ctrl Pts',(-0.929503603080839,2.48192374326381,
45.6942306077308));
#61338=CARTESIAN_POINT('Ctrl Pts',(-1.48294296488667,2.53254694014243,45.6943635436273));
#61339=CARTESIAN_POINT('Ctrl Pts',(-1.84923144734727,2.58285611046353,45.6951271660723));
#61340=CARTESIAN_POINT('Ctrl Pts',(-2.58528683030832,2.71814578051949,45.6960725289316));
#61341=CARTESIAN_POINT('Ctrl Pts',(-2.95437944818565,2.80386392547483,45.695959587621));
#61342=CARTESIAN_POINT('Ctrl Pts',(-3.66834194740326,3.00499350179398,45.695870963165));
#61343=CARTESIAN_POINT('Ctrl Pts',(-4.01319449081232,3.11891878356932,45.696));
#61344=CARTESIAN_POINT('Ctrl Pts',(-4.35247056279534,3.248,45.696));
#61345=CARTESIAN_POINT('Origin',(-12.256,29.392,39.968));
#61346=CARTESIAN_POINT('Origin',(-12.256,29.392,39.968));
#61347=CARTESIAN_POINT('Ctrl Pts',(4.39516096358101,3.27057537586253,45.695842677698));
#61348=CARTESIAN_POINT('Ctrl Pts',(3.10136038026502,2.76989103636905,45.6999183484526));
#61349=CARTESIAN_POINT('Ctrl Pts',(1.55459125658799,2.44759664360609,45.6978772609464));
#61350=CARTESIAN_POINT('Ctrl Pts',(0.00845534674966224,2.44800610805417,
45.696010238955));
#61351=CARTESIAN_POINT('Ctrl Pts',(0.00423047718001614,2.448,45.6960051189726));
#61352=CARTESIAN_POINT('Ctrl Pts',(7.47837257143373E-16,2.448,45.696));
#61353=CARTESIAN_POINT('Ctrl Pts',(4.39511536874253,3.02604293559063,45.7030390251783));
#61354=CARTESIAN_POINT('Ctrl Pts',(3.10299573355848,2.61832690373019,45.5463077383758));
#61355=CARTESIAN_POINT('Ctrl Pts',(1.53064193566912,2.45080363107014,45.6242176396158));
#61356=CARTESIAN_POINT('Ctrl Pts',(0.00835778454095319,2.4479978870276,
45.6956086270239));
#61357=CARTESIAN_POINT('Ctrl Pts',(0.00417737580197284,2.448,45.695804314302));
#61358=CARTESIAN_POINT('Ctrl Pts',(7.47837257143373E-16,2.448,45.696));
#61359=CARTESIAN_POINT('Ctrl Pts',(4.39671743528037,2.59903454561625,45.5050418831425));
#61360=CARTESIAN_POINT('Ctrl Pts',(3.05527533000142,2.47592075525703,45.2585583869767));
#61361=CARTESIAN_POINT('Ctrl Pts',(1.49436708678789,2.44969437712917,45.4997611979407));
#61362=CARTESIAN_POINT('Ctrl Pts',(0.00817708117964293,2.44799748268289,
45.6949007347785));
#61363=CARTESIAN_POINT('Ctrl Pts',(0.00408478680943832,2.448,45.6954541858716));
#61364=CARTESIAN_POINT('Ctrl Pts',(7.47837257143373E-16,2.448,45.696));
#61365=CARTESIAN_POINT('Ctrl Pts',(4.4000397197984,2.44795709552943,45.0779870733328));
#61366=CARTESIAN_POINT('Ctrl Pts',(2.95581829667796,2.4492887212198,44.9980915455101));
#61367=CARTESIAN_POINT('Ctrl Pts',(1.46391650084949,2.4480041008596,45.3714533842438));
#61368=CARTESIAN_POINT('Ctrl Pts',(0.00798512064170265,2.44799999699524,
45.6942002504552));
#61369=CARTESIAN_POINT('Ctrl Pts',(0.00399219781690372,2.448,45.6951040574412));
#61370=CARTESIAN_POINT('Ctrl Pts',(7.47837257143373E-16,2.448,45.696));
#61371=CARTESIAN_POINT('Ctrl Pts',(4.40145261138498,2.448,44.8961576078484));
#61372=CARTESIAN_POINT('Ctrl Pts',(2.91352207632623,2.448,44.8865642443111));
#61373=CARTESIAN_POINT('Ctrl Pts',(1.45091428114908,2.44799999999988,45.3167261493743));
#61374=CARTESIAN_POINT('Ctrl Pts',(0.00790328288195149,2.448,45.6939015162397));
#61375=CARTESIAN_POINT('Ctrl Pts',(0.00395271020241243,2.448,45.6949547336815));
#61376=CARTESIAN_POINT('Ctrl Pts',(7.47837257143373E-16,2.448,45.696));
#61377=CARTESIAN_POINT('',(0.113153243773417,2.44852303636207,45.696));
#61378=CARTESIAN_POINT('Origin',(0.,14.688,45.696));
#61379=CARTESIAN_POINT('Origin',(0.,14.688,45.696));
#61380=CARTESIAN_POINT('Ctrl Pts',(7.46282150093834E-16,2.448,45.696));
#61381=CARTESIAN_POINT('Ctrl Pts',(0.00395271020241243,2.448,45.6949547336815));
#61382=CARTESIAN_POINT('Ctrl Pts',(0.00790328288195149,2.448,45.6939015162397));
#61383=CARTESIAN_POINT('Ctrl Pts',(1.43512030035333,2.44799999999988,45.320854392685));
#61384=CARTESIAN_POINT('Ctrl Pts',(2.88141996176407,2.448,44.896));
#61385=CARTESIAN_POINT('Ctrl Pts',(4.35247056279534,2.448,44.896));
#61386=CARTESIAN_POINT('Origin',(16.744,3.248,39.968));
#61387=CARTESIAN_POINT('Origin',(16.744,3.248,39.968));
#61388=CARTESIAN_POINT('Origin',(13.056,22.032,45.696));
#61389=CARTESIAN_POINT('',(13.056,22.032,44.064));
#61390=CARTESIAN_POINT('Origin',(0.,2.448,42.432));
#61391=CARTESIAN_POINT('',(8.772,2.448,39.968));
#61392=CARTESIAN_POINT('',(-6.528,2.448,40.332));
#61393=CARTESIAN_POINT('Origin',(-6.528,2.448,42.432));
#61394=CARTESIAN_POINT('',(6.528,2.448,40.332));
#61395=CARTESIAN_POINT('Origin',(6.528,2.448,42.432));
#61396=CARTESIAN_POINT('Origin',(-17.544,2.448,39.168));
#61397=CARTESIAN_POINT('',(-17.544,2.448,39.968));
#61398=CARTESIAN_POINT('Origin',(-16.744,2.448,39.968));
#61399=CARTESIAN_POINT('',(-16.744,2.448,39.168));
#61400=CARTESIAN_POINT('Origin',(17.544,2.448,45.696));
#61401=CARTESIAN_POINT('Origin',(0.,30.192,42.432));
#61402=CARTESIAN_POINT('Origin',(8.772,3.248,39.968));
#61403=CARTESIAN_POINT('',(8.772,3.248,39.168));
#61404=CARTESIAN_POINT('Origin',(8.772,21.232,39.968));
#61405=CARTESIAN_POINT('',(-13.056,22.032,39.968));
#61406=CARTESIAN_POINT('',(8.772,22.032,39.968));
#61407=CARTESIAN_POINT('',(-12.256,21.232,39.168));
#61408=CARTESIAN_POINT('Origin',(-12.256,21.232,39.968));
#61409=CARTESIAN_POINT('',(8.772,21.232,39.168));
#61410=CARTESIAN_POINT('Origin',(-12.256,12.24,39.968));
#61411=CARTESIAN_POINT('',(-12.256,12.24,39.168));
#61412=CARTESIAN_POINT('',(-13.056,12.24,39.968));
#61413=CARTESIAN_POINT('Origin',(0.,22.032,42.432));
#61414=CARTESIAN_POINT('',(-13.056,22.032,40.8));
#61415=CARTESIAN_POINT('Origin',(0.,14.688,46.3872037037125));
#61416=CARTESIAN_POINT('',(-5.7528,14.688,46.3872037037125));
#61417=CARTESIAN_POINT('Origin',(0.,14.688,46.3872037037125));
#61418=CARTESIAN_POINT('',(-6.3648,14.688,47.1648));
#61419=CARTESIAN_POINT('Origin',(-6.5528,14.688,46.3872037037125));
#61420=CARTESIAN_POINT('Origin',(0.,14.688,47.1648));
#61421=CARTESIAN_POINT('Origin',(0.,14.688,40.7184));
#61422=CARTESIAN_POINT('',(-5.7528,14.688,40.7184));
#61423=CARTESIAN_POINT('Origin',(0.,14.688,40.7184));
#61424=CARTESIAN_POINT('',(-5.7528,14.688,40.7184));
#61425=CARTESIAN_POINT('Origin',(0.,14.688,46.6912));
#61426=CARTESIAN_POINT('',(-11.44,14.688,47.4912));
#61427=CARTESIAN_POINT('Origin',(0.,14.688,47.4912));
#61428=CARTESIAN_POINT('',(-12.24,14.688,46.6912));
#61429=CARTESIAN_POINT('Origin',(-11.44,14.688,46.6912));
#61430=CARTESIAN_POINT('Origin',(0.,14.688,46.6912));
#61431=CARTESIAN_POINT('Origin',(0.,14.688,47.4912));
#61432=CARTESIAN_POINT('',(11.3943409947345,14.688,47.4912));
#61433=CARTESIAN_POINT('Origin',(0.,14.688,47.4912));
#61434=CARTESIAN_POINT('Origin',(0.,14.688,45.696));
#61435=CARTESIAN_POINT('',(-12.24,14.688,45.696));
#61436=CARTESIAN_POINT('',(-12.24,14.688,45.696));
#61437=CARTESIAN_POINT('',(-4.59359814877846,3.34267250153002,45.696));
#61438=CARTESIAN_POINT('Origin',(0.,14.688,45.696));
#61439=CARTESIAN_POINT('Origin',(0.,14.688,45.696));
#61440=CARTESIAN_POINT('',(4.59359814877845,3.34267250153002,45.696));
#61441=CARTESIAN_POINT('Origin',(0.,14.688,45.696));
#61442=CARTESIAN_POINT('',(10.4030656451586,21.13732749847,45.696));
#61443=CARTESIAN_POINT('Origin',(0.,14.688,45.696));
#61444=CARTESIAN_POINT('',(-10.4030656451586,21.13732749847,45.696));
#61445=CARTESIAN_POINT('Origin',(0.,14.688,45.696));
#61446=CARTESIAN_POINT('Origin',(0.,14.688,45.696));
#61447=CARTESIAN_POINT('Origin',(0.,14.688,46.6912));
#61448=CARTESIAN_POINT('',(10.608,14.688,46.8384));
#61449=CARTESIAN_POINT('Origin',(0.,14.688,46.8384));
#61450=CARTESIAN_POINT('Origin',(11.3943409947345,14.688,46.6912));
#61451=CARTESIAN_POINT('Origin',(6.528,3.248,42.432));
#61452=CARTESIAN_POINT('',(6.528,3.248,41.132));
#61453=CARTESIAN_POINT('Origin',(6.528,3.248,40.332));
#61454=CARTESIAN_POINT('',(5.228,3.248,42.432));
#61455=CARTESIAN_POINT('Origin',(6.528,3.248,42.432));
#61456=CARTESIAN_POINT('Origin',(6.528,3.248,42.432));
#61457=CARTESIAN_POINT('Origin',(6.528,2.448,42.432));
#61458=CARTESIAN_POINT('',(5.228,6.12,42.432));
#61459=CARTESIAN_POINT('',(5.228,2.448,42.432));
#61460=CARTESIAN_POINT('Origin',(6.528,6.12,42.432));
#61461=CARTESIAN_POINT('Origin',(-6.528,3.248,42.432));
#61462=CARTESIAN_POINT('',(-6.528,3.248,41.132));
#61463=CARTESIAN_POINT('Origin',(-6.528,3.248,40.332));
#61464=CARTESIAN_POINT('',(-7.828,3.248,42.432));
#61465=CARTESIAN_POINT('Origin',(-6.528,3.248,42.432));
#61466=CARTESIAN_POINT('Origin',(-6.528,3.248,42.432));
#61467=CARTESIAN_POINT('Origin',(-6.528,2.448,42.432));
#61468=CARTESIAN_POINT('',(-7.828,6.12,42.432));
#61469=CARTESIAN_POINT('',(-7.828,2.448,42.432));
#61470=CARTESIAN_POINT('Origin',(-6.528,6.12,42.432));
#61471=CARTESIAN_POINT('Origin',(-16.64932749847,20.4,44.896));
#61472=CARTESIAN_POINT('',(-16.64932749847,21.13732749847,45.696));
#61473=CARTESIAN_POINT('',(-16.64932749847,3.34267250153002,45.696));
#61474=CARTESIAN_POINT('',(-16.64932749847,20.4,45.696));
#61475=CARTESIAN_POINT('',(-15.912,4.08,45.2064));
#61476=CARTESIAN_POINT('Origin',(-16.64932749847,3.34267250153002,44.896));
#61477=CARTESIAN_POINT('',(-15.912,20.4,45.2064));
#61478=CARTESIAN_POINT('',(-15.912,20.4,45.2064));
#61479=CARTESIAN_POINT('Origin',(-16.64932749847,21.13732749847,44.896));
#61480=CARTESIAN_POINT('Origin',(-15.912,3.34267250153002,44.896));
#61481=CARTESIAN_POINT('',(-6.88783275058274,4.08000000000001,45.2064));
#61482=CARTESIAN_POINT('Ctrl Pts',(-6.88783275058276,4.08,45.2064));
#61483=CARTESIAN_POINT('Ctrl Pts',(-6.83096980964154,4.0598235620632,45.2543273276803));
#61484=CARTESIAN_POINT('Ctrl Pts',(-6.7651197403416,4.03741502983645,45.2945582388546));
#61485=CARTESIAN_POINT('Ctrl Pts',(-6.39957290725477,3.9155905586413,45.4848436925738));
#61486=CARTESIAN_POINT('Ctrl Pts',(-5.98530408411679,3.7896019396787,45.564325669844));
#61487=CARTESIAN_POINT('Ctrl Pts',(-5.5447169847327,3.65682068790766,45.635102112391));
#61488=CARTESIAN_POINT('Ctrl Pts',(-5.32942559902382,3.59265625235564,45.6587020324601));
#61489=CARTESIAN_POINT('Ctrl Pts',(-5.01397139988192,3.49312899095025,45.6826190067178));
#61490=CARTESIAN_POINT('Ctrl Pts',(-4.89575271613861,3.45453624015517,45.6891574202889));
#61491=CARTESIAN_POINT('Ctrl Pts',(-4.74288425804082,3.40004644173792,45.694072800358));
#61492=CARTESIAN_POINT('Ctrl Pts',(-4.70238437966304,3.38513990705534,45.6950176500099));
#61493=CARTESIAN_POINT('Ctrl Pts',(-4.63941311517471,3.36096086412175,45.6958408853381));
#61494=CARTESIAN_POINT('Ctrl Pts',(-4.61634398319733,3.35188203936778,45.696));
#61495=CARTESIAN_POINT('Ctrl Pts',(-4.59359814877846,3.34267250153002,45.696));
#61496=CARTESIAN_POINT('',(-15.912,4.08,45.2064));
#61497=CARTESIAN_POINT('',(-15.912,3.34267250153002,45.696));
#61498=CARTESIAN_POINT('Origin',(15.912,21.13732749847,44.896));
#61499=CARTESIAN_POINT('',(-11.2847224157265,20.4,45.2064));
#61500=CARTESIAN_POINT('Ctrl Pts',(-10.4030656451586,21.13732749847,45.696));
#61501=CARTESIAN_POINT('Ctrl Pts',(-10.4051770230818,21.1339217475383,45.696));
#61502=CARTESIAN_POINT('Ctrl Pts',(-10.4073411793795,21.1305091350682,45.6959782528326));
#61503=CARTESIAN_POINT('Ctrl Pts',(-10.412554449671,21.1224696164265,45.6958753597619));
#61504=CARTESIAN_POINT('Ctrl Pts',(-10.4156410384128,21.1178470255194,45.6957761688512));
#61505=CARTESIAN_POINT('Ctrl Pts',(-10.4269111127494,21.101439194627,45.6952815482675));
#61506=CARTESIAN_POINT('Ctrl Pts',(-10.4354731270868,21.0898118955789,45.6946703826387));
#61507=CARTESIAN_POINT('Ctrl Pts',(-10.5276360945525,20.9718731085772,45.6859518637731));
#61508=CARTESIAN_POINT('Ctrl Pts',(-10.6546192820411,20.8677270702112,45.6569089689747));
#61509=CARTESIAN_POINT('Ctrl Pts',(-10.8999196049235,20.6799375325347,45.5604011294049));
#61510=CARTESIAN_POINT('Ctrl Pts',(-11.0271541759068,20.5894785071695,45.4916387532884));
#61511=CARTESIAN_POINT('Ctrl Pts',(-11.189723388502,20.4714505593328,45.3443731595757));
#61512=CARTESIAN_POINT('Ctrl Pts',(-11.2432877828146,20.4321606305034,45.2821292970099));
#61513=CARTESIAN_POINT('Ctrl Pts',(-11.2838716320031,20.400661136201,45.2079669722959));
#61514=CARTESIAN_POINT('Ctrl Pts',(-11.284297802453,20.4003300968063,45.2071841155039));
#61515=CARTESIAN_POINT('Ctrl Pts',(-11.2847224157265,20.4,45.2064));
#61516=CARTESIAN_POINT('',(15.912,21.13732749847,45.696));
#61517=CARTESIAN_POINT('',(15.912,20.4,45.2064));
#61518=CARTESIAN_POINT('Origin',(0.,14.688,44.9814350779728));
#61519=CARTESIAN_POINT('Origin',(0.,14.688,45.2064));
#61520=CARTESIAN_POINT('Origin',(0.,14.688,44.9814350779728));
#61521=CARTESIAN_POINT('',(6.88783275058272,4.08,45.2064));
#61522=CARTESIAN_POINT('Ctrl Pts',(6.88783275058275,4.07999999999999,45.2064));
#61523=CARTESIAN_POINT('Ctrl Pts',(6.81886324438962,4.05552784048444,45.2645314309206));
#61524=CARTESIAN_POINT('Ctrl Pts',(6.73479715088626,4.02711895305195,45.3128039443106));
#61525=CARTESIAN_POINT('Ctrl Pts',(6.37658245357399,3.90895311670654,45.4835230174535));
#61526=CARTESIAN_POINT('Ctrl Pts',(6.01691030549754,3.79918184362475,45.5580047227756));
#61527=CARTESIAN_POINT('Ctrl Pts',(5.4669145728647,3.63330799139618,45.6490772612781));
#61528=CARTESIAN_POINT('Ctrl Pts',(5.1442770940251,3.53803359519506,45.6769668597336));
#61529=CARTESIAN_POINT('Ctrl Pts',(4.82263423748175,3.42860301313298,45.6916369428731));
#61530=CARTESIAN_POINT('Ctrl Pts',(4.76176127218778,3.40713850397811,45.6937147455139));
#61531=CARTESIAN_POINT('Ctrl Pts',(4.67424460245221,3.37441113690961,45.6954366167826));
#61532=CARTESIAN_POINT('Ctrl Pts',(4.64655042016146,3.36378090096371,45.695796654937));
#61533=CARTESIAN_POINT('Ctrl Pts',(4.61048568759284,3.34947405358982,45.6959780669794));
#61534=CARTESIAN_POINT('Ctrl Pts',(4.60204627195492,3.34609305355812,45.696));
#61535=CARTESIAN_POINT('Ctrl Pts',(4.59359814877844,3.34267250153004,45.696));
#61536=CARTESIAN_POINT('',(11.2847224157265,20.4,45.2064));
#61537=CARTESIAN_POINT('Origin',(0.,14.688,45.2064));
#61538=CARTESIAN_POINT('Ctrl Pts',(10.4030656451586,21.13732749847,45.696));
#61539=CARTESIAN_POINT('Ctrl Pts',(10.4034528587117,21.1367029049737,45.696));
#61540=CARTESIAN_POINT('Ctrl Pts',(10.4038419091445,21.1360779805853,45.6959992685327));
#61541=CARTESIAN_POINT('Ctrl Pts',(10.4067993400092,21.1313473906548,45.6959881825164));
#61542=CARTESIAN_POINT('Ctrl Pts',(10.409442322896,21.1272325286132,45.6959469405597));
#61543=CARTESIAN_POINT('Ctrl Pts',(10.4165444903014,21.1164637513178,45.6957555036594));
#61544=CARTESIAN_POINT('Ctrl Pts',(10.4210983853722,21.1098376988435,45.6955548983378));
#61545=CARTESIAN_POINT('Ctrl Pts',(10.4423960109042,21.0800225292309,45.6942830109848));
#61546=CARTESIAN_POINT('Ctrl Pts',(10.4606745049416,21.0575445714608,45.6923105556957));
#61547=CARTESIAN_POINT('Ctrl Pts',(10.5332222285603,20.9760257865206,45.6818919339335));
#61548=CARTESIAN_POINT('Ctrl Pts',(10.5968068470649,20.9192489972096,45.6676377403279));
#61549=CARTESIAN_POINT('Ctrl Pts',(10.7768228876743,20.7700779575399,45.6142654321202));
#61550=CARTESIAN_POINT('Ctrl Pts',(10.9210832070263,20.6659568730065,45.5556873871454));
#61551=CARTESIAN_POINT('Ctrl Pts',(11.1395119114092,20.5079861571895,45.398243288761));
#61552=CARTESIAN_POINT('Ctrl Pts',(11.2127184779424,20.4549727268256,45.3235592719424));
#61553=CARTESIAN_POINT('Ctrl Pts',(11.2716513432665,20.4101014026675,45.2296098269067));
#61554=CARTESIAN_POINT('Ctrl Pts',(11.2783609804129,20.404945416479,45.2181473954941));
#61555=CARTESIAN_POINT('Ctrl Pts',(11.2847224157265,20.4,45.2064));
#61556=CARTESIAN_POINT('Origin',(-17.544,2.448,45.696));
#61557=CARTESIAN_POINT('',(16.64932749847,21.13732749847,45.696));
#61558=CARTESIAN_POINT('',(15.912,21.13732749847,45.696));
#61559=CARTESIAN_POINT('',(16.64932749847,3.34267250153002,45.696));
#61560=CARTESIAN_POINT('',(16.64932749847,4.08,45.696));
#61561=CARTESIAN_POINT('',(-15.912,3.34267250153002,45.696));
#61562=CARTESIAN_POINT('Origin',(-15.912,3.34267250153002,44.896));
#61563=CARTESIAN_POINT('',(15.912,4.08,45.2064));
#61564=CARTESIAN_POINT('Origin',(16.64932749847,3.34267250153002,44.896));
#61565=CARTESIAN_POINT('',(-15.912,4.08,45.2064));
#61566=CARTESIAN_POINT('Origin',(15.912,21.13732749847,44.896));
#61567=CARTESIAN_POINT('',(15.912,20.4,45.2064));
#61568=CARTESIAN_POINT('',(15.912,20.4,45.2064));
#61569=CARTESIAN_POINT('Origin',(16.64932749847,21.13732749847,44.896));
#61570=CARTESIAN_POINT('Origin',(16.64932749847,4.08,44.896));
#61571=CARTESIAN_POINT('',(15.912,4.08,45.2064));
#61572=CARTESIAN_POINT('Origin',(-14.28,5.712,44.4064));
#61573=CARTESIAN_POINT('',(-13.6272,5.712,45.0432));
#61574=CARTESIAN_POINT('Origin',(-14.28,5.712,45.0432));
#61575=CARTESIAN_POINT('',(-13.1429627027995,5.712,45.2064));
#61576=CARTESIAN_POINT('Origin',(-13.1429627027995,5.712,44.4064));
#61577=CARTESIAN_POINT('Origin',(-14.28,5.712,45.2064));
#61578=CARTESIAN_POINT('Origin',(-11.3999163752914,12.24,45.2064));
#61579=CARTESIAN_POINT('',(-13.1429627027995,18.768,45.2064));
#61580=CARTESIAN_POINT('Origin',(-14.28,18.768,45.2064));
#61581=CARTESIAN_POINT('Origin',(-14.28,18.768,44.4064));
#61582=CARTESIAN_POINT('',(-13.6272,18.768,45.0432));
#61583=CARTESIAN_POINT('Origin',(-14.28,18.768,45.0432));
#61584=CARTESIAN_POINT('Origin',(-13.1429627027995,18.768,44.4064));
#61585=CARTESIAN_POINT('Origin',(14.28,5.712,44.4064));
#61586=CARTESIAN_POINT('',(14.9328,5.712,45.0432));
#61587=CARTESIAN_POINT('Origin',(14.28,5.712,45.0432));
#61588=CARTESIAN_POINT('',(15.4170372972005,5.712,45.2064));
#61589=CARTESIAN_POINT('Origin',(15.4170372972005,5.712,44.4064));
#61590=CARTESIAN_POINT('Origin',(14.28,5.712,45.2064));
#61591=CARTESIAN_POINT('Origin',(11.3999163752914,12.24,45.2064));
#61592=CARTESIAN_POINT('',(15.4170372972005,18.768,45.2064));
#61593=CARTESIAN_POINT('Origin',(14.28,18.768,45.2064));
#61594=CARTESIAN_POINT('Origin',(14.28,18.768,44.4064));
#61595=CARTESIAN_POINT('',(14.9328,18.768,45.0432));
#61596=CARTESIAN_POINT('Origin',(14.28,18.768,45.0432));
#61597=CARTESIAN_POINT('Origin',(15.4170372972005,18.768,44.4064));
#61598=CARTESIAN_POINT('Origin',(0.,14.688,46.4864022969699));
#61599=CARTESIAN_POINT('',(8.16,14.688,46.8384));
#61600=CARTESIAN_POINT('Origin',(0.,14.688,46.8384));
#61601=CARTESIAN_POINT('',(7.0176,14.688,47.1648));
#61602=CARTESIAN_POINT('Origin',(7.4416006562771,14.688,46.4864022969699));
#61603=CARTESIAN_POINT('Origin',(0.,14.688,47.1648));
#61604=CARTESIAN_POINT('Origin',(0.,14.688,47.1648));
#61605=CARTESIAN_POINT('Origin',(14.28,18.768,45.0432));
#61606=CARTESIAN_POINT('Origin',(14.28,5.712,45.0432));
#61607=CARTESIAN_POINT('Origin',(-14.28,18.768,45.0432));
#61608=CARTESIAN_POINT('Origin',(-14.28,5.712,45.0432));
#61609=CARTESIAN_POINT('Origin',(-6.528,6.12,42.432));
#61610=CARTESIAN_POINT('Origin',(6.528,6.12,42.432));
#61611=CARTESIAN_POINT('Origin',(0.,14.688,46.8384));
#61612=CARTESIAN_POINT('Origin',(0.,14.688,40.7184));
#61613=CARTESIAN_POINT('',(-3.975,14.688,40.7184));
#61614=CARTESIAN_POINT('Origin',(0.,14.688,40.7184));
#61615=CARTESIAN_POINT('Origin',(0.,14.688,39.268));
#61616=CARTESIAN_POINT('',(-3.975,14.688,39.368));
#61617=CARTESIAN_POINT('Origin',(0.,14.688,39.368));
#61618=CARTESIAN_POINT('',(-4.175,14.688,39.168));
#61619=CARTESIAN_POINT('',(-4.075,14.688,39.268));
#61620=CARTESIAN_POINT('Origin',(0.,14.688,39.168));
#61621=CARTESIAN_POINT('Origin',(0.,14.688,38.352));
#61622=CARTESIAN_POINT('',(-3.975,14.688,38.352));
#61623=CARTESIAN_POINT('Origin',(17.544,2.448,39.168));
#61624=CARTESIAN_POINT('Origin',(-13.056,22.032,39.168));
#61625=CARTESIAN_POINT('Origin',(0.,22.032,42.432));
#99996=UNCERTAINTY_MEASURE_WITH_UNIT(LENGTH_MEASURE(0.01),#100032,
'DISTANCE_ACCURACY_VALUE',
'Maximum model space distance between geometric entities at asserted c
onnectivities');
#100011=UNCERTAINTY_MEASURE_WITH_UNIT(LENGTH_MEASURE(0.01),#100032,
'DISTANCE_ACCURACY_VALUE',
'Maximum model space distance between geometric entities at asserted c
onnectivities');
#100016=(
GEOMETRIC_REPRESENTATION_CONTEXT(3)
GLOBAL_UNCERTAINTY_ASSIGNED_CONTEXT((#99996))
GLOBAL_UNIT_ASSIGNED_CONTEXT((#100032,#100034,#100035))
REPRESENTATION_CONTEXT('','3D')
);
#100031=(
GEOMETRIC_REPRESENTATION_CONTEXT(3)
GLOBAL_UNCERTAINTY_ASSIGNED_CONTEXT((#100011))
GLOBAL_UNIT_ASSIGNED_CONTEXT((#100032,#100034,#100035))
REPRESENTATION_CONTEXT('','3D')
);
#100032=(
LENGTH_UNIT()
NAMED_UNIT(*)
SI_UNIT(.MILLI.,.METRE.)
);
#100034=(
NAMED_UNIT(*)
PLANE_ANGLE_UNIT()
SI_UNIT($,.RADIAN.)
);
#100035=(
NAMED_UNIT(*)
SI_UNIT($,.STERADIAN.)
SOLID_ANGLE_UNIT()
);
#100040=SHAPE_DEFINITION_REPRESENTATION(#100059,#100104);
#100059=PRODUCT_DEFINITION_SHAPE('',$,#100124);
#100104=SHAPE_REPRESENTATION('',(#21261),#100016);
#100119=PRODUCT_DEFINITION_CONTEXT('part definition',#100178,'design');
#100124=PRODUCT_DEFINITION('2026-10-12-11-54-56-863',
'04_Motor_Coupling_Housing',#100143,#100119);
#100143=PRODUCT_DEFINITION_FORMATION('',$,#100184);
#100178=APPLICATION_CONTEXT(
'Core Data for Automotive Mechanical Design Process');
#100179=PRODUCT_CONTEXT('part definition',#100178,'mechanical');
#100184=PRODUCT('2026-10-12-11-54-56-863','04_Motor_Coupling_Housing',$,
(#100179));
#100201=PRESENTATION_STYLE_ASSIGNMENT((#100207));
#100207=SURFACE_STYLE_USAGE(.BOTH.,#100213);
#100213=SURFACE_SIDE_STYLE('',(#100219));
#100219=SURFACE_STYLE_FILL_AREA(#100225);
#100225=FILL_AREA_STYLE('Opaque(20,51,87)',(#100231));
#100231=FILL_AREA_STYLE_COLOUR('Opaque(20,51,87)',#100237);
#100237=COLOUR_RGB('Opaque(20,51,87)',0.0784313725490196,0.2,0.341176470588235);
ENDSEC;
END-ISO-10303-21;
